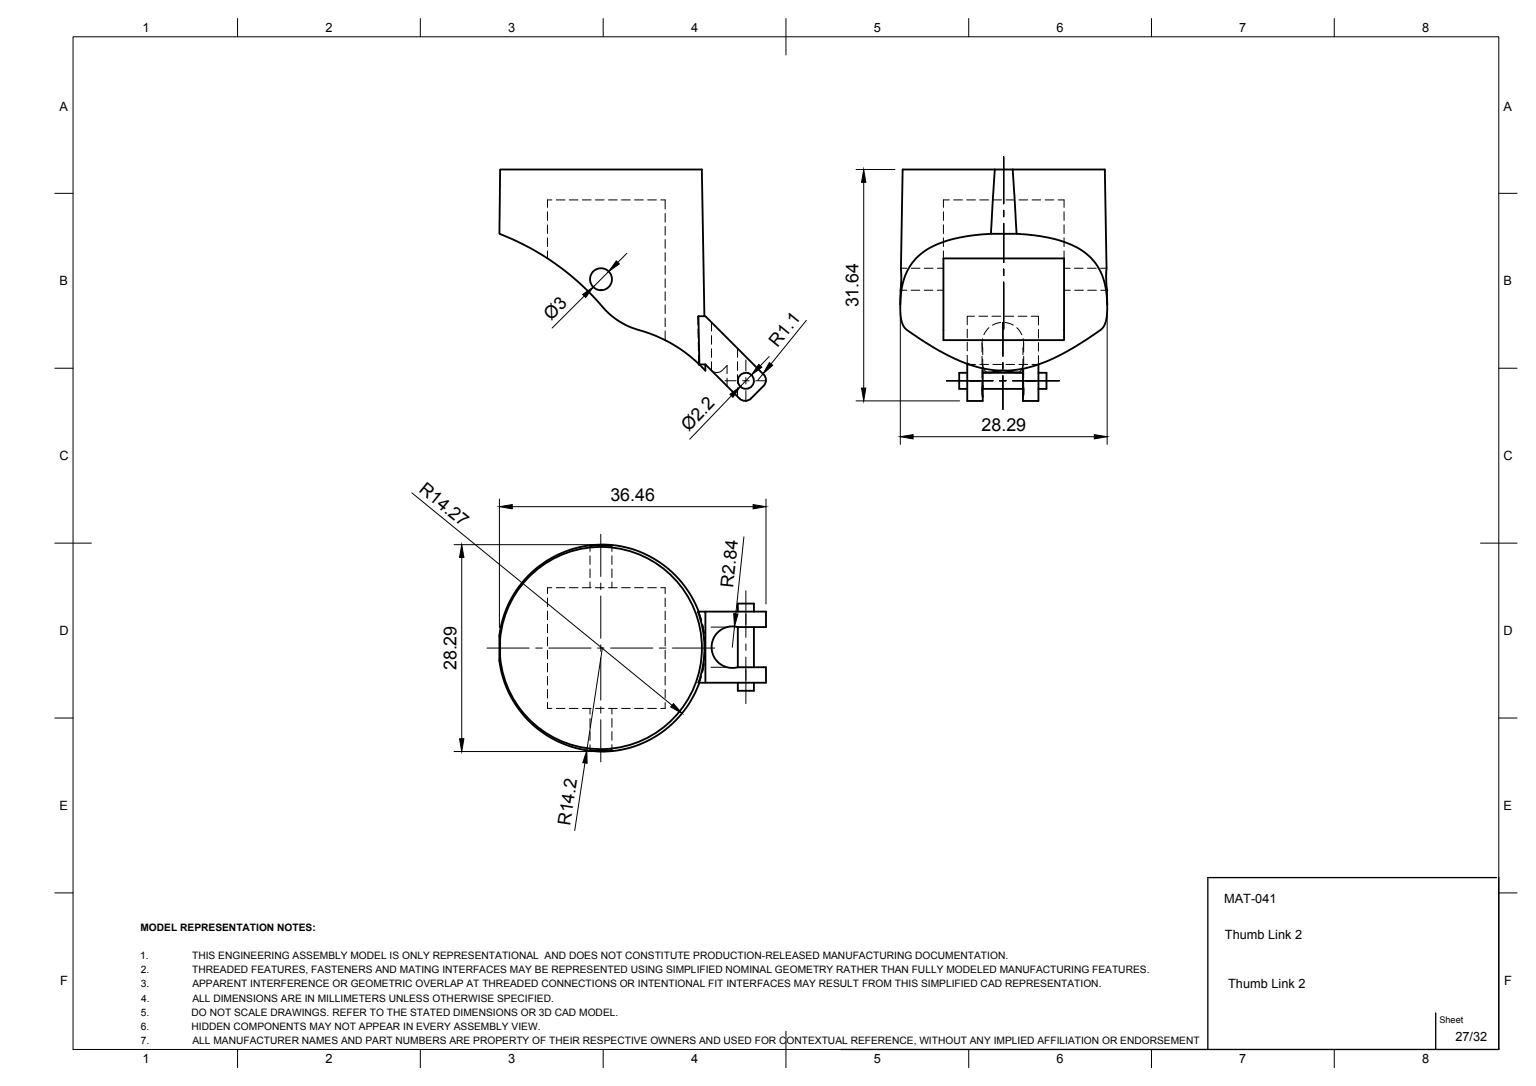
ISO-10303-21;
HEADER;
/* Generated by software containing ST-Developer
 * from STEP Tools, Inc. (www.steptools.com) 
 */

FILE_DESCRIPTION(
/* description */ ('STEP AP214'),
/* implementation_level */ '2;1');

FILE_NAME(
/* name */ 'Thumb Link 2.step',
/* time_stamp */ '2026-11-14T21:57:47-08:00',
/* author */ (''),
/* organization */ (''),
/* preprocessor_version */ 'ST-DEVELOPER v20.2',
/* originating_system */ 'Autodesk Translation Framework v15.17.0.0',
/* authorisation */ '');

FILE_SCHEMA (('AUTOMOTIVE_DESIGN { 1 0 10303 214 3 1 1 }'));
ENDSEC;

DATA;
#10=MECHANICAL_DESIGN_GEOMETRIC_PRESENTATION_REPRESENTATION('',(#262),#13199);
#14=(
BOUNDED_CURVE()
B_SPLINE_CURVE(2,(#12779,#12780,#12781),.UNSPECIFIED.,.F.,.F.)
B_SPLINE_CURVE_WITH_KNOTS((3,3),(-2.71364129597392,-1.62020359036119),
 .UNSPECIFIED.)
CURVE()
GEOMETRIC_REPRESENTATION_ITEM()
RATIONAL_B_SPLINE_CURVE((1.0005626059293,1.00242625759818,1.00269667985146))
REPRESENTATION_ITEM('')
);
#15=(
BOUNDED_CURVE()
B_SPLINE_CURVE(2,(#12785,#12786,#12787),.UNSPECIFIED.,.F.,.F.)
B_SPLINE_CURVE_WITH_KNOTS((3,3),(-1.2490205262323,-0.155582820602816),
 .UNSPECIFIED.)
CURVE()
GEOMETRIC_REPRESENTATION_ITEM()
RATIONAL_B_SPLINE_CURVE((1.00269667985147,1.00242625759819,1.00056260592924))
REPRESENTATION_ITEM('')
);
#16=(
BOUNDED_CURVE()
B_SPLINE_CURVE(2,(#12826,#12827,#12828),.UNSPECIFIED.,.F.,.F.)
B_SPLINE_CURVE_WITH_KNOTS((3,3),(0.587541837462245,1.2406747936684),
 .UNSPECIFIED.)
CURVE()
GEOMETRIC_REPRESENTATION_ITEM()
RATIONAL_B_SPLINE_CURVE((1.00007054095476,1.00010145473128,1.00011392829506))
REPRESENTATION_ITEM('')
);
#124=CONICAL_SURFACE('',#7720,14.3,0.0174532925199433);
#125=CONICAL_SURFACE('',#7729,14.3,0.0174532925199433);
#126=CONICAL_SURFACE('',#7753,14.3,0.0174532925199433);
#199=B_SPLINE_CURVE_WITH_KNOTS('',3,(#12595,#12596,#12597,#12598,#12599,
#12600,#12601,#12602,#12603,#12604,#12605,#12606,#12607,#12608,#12609,#12610,
#12611,#12612,#12613,#12614),.UNSPECIFIED.,.F.,.F.,(4,2,2,2,2,2,2,2,2,4),
(1.13069615346588,1.18716968917911,1.24364799854408,1.30009527290761,1.35654254727113,
1.41319810974912,1.46985367222711,1.526495709458,1.58313774668889,1.58314252031411),
 .UNSPECIFIED.);
#200=B_SPLINE_CURVE_WITH_KNOTS('',3,(#12615,#12616,#12617,#12618,#12619,
#12620,#12621,#12622,#12623,#12624,#12625,#12626,#12627,#12628,#12629,#12630,
#12631,#12632,#12633,#12634,#12635),.UNSPECIFIED.,.F.,.F.,(4,2,2,2,3,2,
2,2,2,4),(0.678287603396378,0.734918137493847,0.791553445216531,0.848204181067131,
0.904854916917731,0.961302354464157,1.01774979201058,1.07422058591236,1.13069137981413,
1.13069615346588),.UNSPECIFIED.);
#201=B_SPLINE_CURVE_WITH_KNOTS('',3,(#12639,#12640,#12641,#12642,#12643,
#12644,#12645,#12646,#12647,#12648,#12649,#12650,#12651,#12652,#12653,#12654,
#12655,#12656,#12657,#12658),.UNSPECIFIED.,.F.,.F.,(4,2,2,2,2,2,2,2,2,4),
(-0.678287603396414,-0.678282829771164,-0.621640792540269,-0.564998755309374,
-0.508343192831388,-0.451687630353401,-0.395240355989875,-0.338793081626349,
-0.282314772261376,-0.225841236548144),.UNSPECIFIED.);
#202=B_SPLINE_CURVE_WITH_KNOTS('',3,(#12662,#12663,#12664,#12665,#12666,
#12667,#12668,#12669,#12670,#12671,#12672,#12673,#12674,#12675,#12676,#12677,
#12678,#12679,#12680,#12681,#12682),.UNSPECIFIED.,.F.,.F.,(4,2,2,2,2,3,
2,2,2,4),(-0.225841236548144,-0.225836462896404,-0.169365668994628,-0.112894875092852,
-0.0564474375464262,0.,0.0566507358506003,0.113301471701201,0.169936779423884,
0.226567313521317),.UNSPECIFIED.);
#203=B_SPLINE_CURVE_WITH_KNOTS('',3,(#12686,#12687,#12688,#12689,#12690,
#12691,#12692,#12693,#12694,#12695,#12696,#12697,#12698,#12699,#12700,#12701,
#12702,#12703),.UNSPECIFIED.,.F.,.F.,(4,2,2,2,2,2,2,2,4),(-0.688543100579729,
-0.654814812371682,-0.585385027074312,-0.486026911248501,-0.386668795422691,
-0.287310679596881,-0.18795256377107,-0.1185227784737,-0.0847944902653396),
 .UNSPECIFIED.);
#204=B_SPLINE_CURVE_WITH_KNOTS('',3,(#12742,#12743,#12744,#12745,#12746,
#12747,#12748,#12749,#12750,#12751),.UNSPECIFIED.,.F.,.F.,(4,2,2,2,4),(2.79683412091131,
2.83278881190682,3.39223982604309,3.96523585047702,4.02795363969691),
 .UNSPECIFIED.);
#205=B_SPLINE_CURVE_WITH_KNOTS('',3,(#12753,#12754,#12755,#12756,#12757,
#12758,#12759,#12760,#12761,#12762),.UNSPECIFIED.,.F.,.F.,(4,2,2,2,4),(10.3179905566208,
10.457151700737,10.6290799698098,10.8010082388826,10.8999538958969),
 .UNSPECIFIED.);
#206=B_SPLINE_CURVE_WITH_KNOTS('',3,(#12764,#12765,#12766,#12767,#12768,
#12769,#12770,#12771,#12772,#12773,#12774,#12775,#12776,#12777),
 .UNSPECIFIED.,.F.,.F.,(4,2,2,2,2,2,4),(-7.02551957351303,-6.83439163802274,
-6.07684267508665,-5.67712314178527,-5.27740360848388,-4.91546143594968,
-4.72326894801671),.UNSPECIFIED.);
#207=B_SPLINE_CURVE_WITH_KNOTS('',3,(#12789,#12790,#12791,#12792,#12793,
#12794,#12795,#12796,#12797,#12798,#12799,#12800,#12801,#12802),
 .UNSPECIFIED.,.F.,.F.,(4,2,2,2,2,2,4),(-4.38376957881428,-4.1915770908813,
-3.82963491834711,-3.42991538504572,-3.03019585174433,-2.27264688880825,
-2.08151895331795),.UNSPECIFIED.);
#208=B_SPLINE_CURVE_WITH_KNOTS('',3,(#12804,#12805,#12806,#12807,#12808,
#12809,#12810,#12811,#12812,#12813),.UNSPECIFIED.,.F.,.F.,(4,2,2,2,4),(6.41116921174888,
6.5101148687632,6.68204313783601,6.85397140690883,6.993132551025),
 .UNSPECIFIED.);
#209=B_SPLINE_CURVE_WITH_KNOTS('',3,(#12815,#12816,#12817,#12818,#12819,
#12820,#12821,#12822,#12823,#12824),.UNSPECIFIED.,.F.,.F.,(4,2,2,2,4),(5.02250397090605,
5.11122789934489,5.68422392377882,6.24367493791509,6.2796296289106),
 .UNSPECIFIED.);
#210=B_SPLINE_CURVE_WITH_KNOTS('',3,(#12831,#12832,#12833,#12834,#12835),
 .UNSPECIFIED.,.F.,.F.,(4,1,4),(0.0247143916721011,0.0279654930527155,0.0312302909052024),
 .UNSPECIFIED.);
#211=B_SPLINE_CURVE_WITH_KNOTS('',3,(#12862,#12863,#12864,#12865,#12866,
#12867,#12868,#12869,#12870,#12871),.UNSPECIFIED.,.F.,.F.,(4,2,2,2,4),(4.05396350737764,
4.25173386269399,4.53823187491096,4.82472988712792,5.02250024244427),
 .UNSPECIFIED.);
#226=SHAPE_REPRESENTATION_RELATIONSHIP('SRR','None',#13298,#244);
#244=ADVANCED_BREP_SHAPE_REPRESENTATION('',(#280),#13194);
#262=STYLED_ITEM('',(#13409),#280);
#280=MANIFOLD_SOLID_BREP('Body1',#6857);
#368=FACE_BOUND('',#2609,.T.);
#369=FACE_BOUND('',#2610,.T.);
#370=FACE_BOUND('',#2620,.T.);
#371=FACE_BOUND('',#2622,.T.);
#372=FACE_BOUND('',#2626,.T.);
#373=FACE_BOUND('',#2629,.T.);
#374=FACE_BOUND('',#2636,.T.);
#375=FACE_BOUND('',#2638,.T.);
#392=ELLIPSE('',#7706,4.01857269385652,2.84156000250712);
#393=ELLIPSE('',#7707,4.01857269388513,2.84156000253857);
#394=ELLIPSE('',#7708,4.01857269388335,2.841560002536);
#395=ELLIPSE('',#7709,4.01857269388599,2.84156000253982);
#396=ELLIPSE('',#7710,4.01857269402875,2.84156000270659);
#573=PLANE('',#7723);
#574=PLANE('',#7724);
#575=PLANE('',#7726);
#576=PLANE('',#7728);
#577=PLANE('',#7735);
#578=PLANE('',#7736);
#579=PLANE('',#7737);
#580=PLANE('',#7740);
#581=PLANE('',#7743);
#582=PLANE('',#7744);
#583=PLANE('',#7746);
#584=PLANE('',#7749);
#585=PLANE('',#7750);
#586=PLANE('',#7754);
#587=PLANE('',#7755);
#588=PLANE('',#7756);
#589=PLANE('',#7757);
#590=PLANE('',#7758);
#591=PLANE('',#7761);
#592=PLANE('',#7764);
#593=PLANE('',#7765);
#594=PLANE('',#7772);
#595=PLANE('',#7773);
#1044=LINE('',#12593,#1562);
#1045=LINE('',#12660,#1563);
#1046=LINE('',#12707,#1564);
#1047=LINE('',#12711,#1565);
#1048=LINE('',#12715,#1566);
#1049=LINE('',#12719,#1567);
#1050=LINE('',#12725,#1568);
#1051=LINE('',#12731,#1569);
#1052=LINE('',#12737,#1570);
#1053=LINE('',#12838,#1571);
#1054=LINE('',#12839,#1572);
#1055=LINE('',#12842,#1573);
#1056=LINE('',#12846,#1574);
#1057=LINE('',#12848,#1575);
#1058=LINE('',#12853,#1576);
#1059=LINE('',#12855,#1577);
#1060=LINE('',#12857,#1578);
#1061=LINE('',#12858,#1579);
#1062=LINE('',#12876,#1580);
#1063=LINE('',#12879,#1581);
#1064=LINE('',#12882,#1582);
#1065=LINE('',#12884,#1583);
#1066=LINE('',#12885,#1584);
#1067=LINE('',#12893,#1585);
#1068=LINE('',#12895,#1586);
#1069=LINE('',#12896,#1587);
#1070=LINE('',#12903,#1588);
#1071=LINE('',#12905,#1589);
#1072=LINE('',#12906,#1590);
#1073=LINE('',#12908,#1591);
#1074=LINE('',#12913,#1592);
#1075=LINE('',#12915,#1593);
#1076=LINE('',#12916,#1594);
#1077=LINE('',#12920,#1595);
#1078=LINE('',#12924,#1596);
#1079=LINE('',#12925,#1597);
#1080=LINE('',#12927,#1598);
#1081=LINE('',#12931,#1599);
#1082=LINE('',#12932,#1600);
#1083=LINE('',#12935,#1601);
#1084=LINE('',#12939,#1602);
#1085=LINE('',#12940,#1603);
#1086=LINE('',#12944,#1604);
#1087=LINE('',#12945,#1605);
#1088=LINE('',#12947,#1606);
#1089=LINE('',#12948,#1607);
#1090=LINE('',#12949,#1608);
#1091=LINE('',#12952,#1609);
#1092=LINE('',#12954,#1610);
#1093=LINE('',#12955,#1611);
#1094=LINE('',#12956,#1612);
#1095=LINE('',#12960,#1613);
#1096=LINE('',#12961,#1614);
#1097=LINE('',#12962,#1615);
#1098=LINE('',#12964,#1616);
#1099=LINE('',#12979,#1617);
#1100=LINE('',#12980,#1618);
#1101=LINE('',#12981,#1619);
#1102=LINE('',#12983,#1620);
#1562=VECTOR('',#9549,1.5);
#1563=VECTOR('',#9552,1.5);
#1564=VECTOR('',#9559,1000.);
#1565=VECTOR('',#9562,1000.);
#1566=VECTOR('',#9565,1000.);
#1567=VECTOR('',#9568,1000.);
#1568=VECTOR('',#9575,1.1);
#1569=VECTOR('',#9582,1.1);
#1570=VECTOR('',#9589,1.1);
#1571=VECTOR('',#9600,1000.);
#1572=VECTOR('',#9601,1000.);
#1573=VECTOR('',#9604,1000.);
#1574=VECTOR('',#9609,1000.);
#1575=VECTOR('',#9610,1000.);
#1576=VECTOR('',#9615,1000.);
#1577=VECTOR('',#9616,1000.);
#1578=VECTOR('',#9617,1000.);
#1579=VECTOR('',#9618,1000.);
#1580=VECTOR('',#9627,1000.);
#1581=VECTOR('',#9630,1000.);
#1582=VECTOR('',#9633,1000.);
#1583=VECTOR('',#9636,1000.);
#1584=VECTOR('',#9637,1000.);
#1585=VECTOR('',#9646,1000.);
#1586=VECTOR('',#9647,1000.);
#1587=VECTOR('',#9648,1000.);
#1588=VECTOR('',#9655,1000.);
#1589=VECTOR('',#9656,1000.);
#1590=VECTOR('',#9657,1000.);
#1591=VECTOR('',#9660,1000.);
#1592=VECTOR('',#9665,1000.);
#1593=VECTOR('',#9666,1000.);
#1594=VECTOR('',#9667,1000.);
#1595=VECTOR('',#9670,1000.);
#1596=VECTOR('',#9673,1000.);
#1597=VECTOR('',#9674,1000.);
#1598=VECTOR('',#9675,1000.);
#1599=VECTOR('',#9680,1000.);
#1600=VECTOR('',#9681,1000.);
#1601=VECTOR('',#9684,1000.);
#1602=VECTOR('',#9689,1000.);
#1603=VECTOR('',#9690,10.);
#1604=VECTOR('',#9695,1000.);
#1605=VECTOR('',#9696,1000.);
#1606=VECTOR('',#9697,1000.);
#1607=VECTOR('',#9698,1000.);
#1608=VECTOR('',#9699,1000.);
#1609=VECTOR('',#9702,1000.);
#1610=VECTOR('',#9703,1000.);
#1611=VECTOR('',#9704,1000.);
#1612=VECTOR('',#9705,1000.);
#1613=VECTOR('',#9708,1000.);
#1614=VECTOR('',#9709,1000.);
#1615=VECTOR('',#9710,1000.);
#1616=VECTOR('',#9713,1000.);
#1617=VECTOR('',#9742,1000.);
#1618=VECTOR('',#9743,1000.);
#1619=VECTOR('',#9744,1000.);
#1620=VECTOR('',#9747,1000.);
#1767=CYLINDRICAL_SURFACE('',#7701,1.5);
#1768=CYLINDRICAL_SURFACE('',#7703,1.5);
#1769=CYLINDRICAL_SURFACE('',#7705,2.84156000253601);
#1770=CYLINDRICAL_SURFACE('',#7711,1.1);
#1771=CYLINDRICAL_SURFACE('',#7714,1.1);
#1772=CYLINDRICAL_SURFACE('',#7717,1.1);
#1773=CYLINDRICAL_SURFACE('',#7731,19.25);
#1774=CYLINDRICAL_SURFACE('',#7766,1.1);
#1775=CYLINDRICAL_SURFACE('',#7767,1.1);
#1776=CYLINDRICAL_SURFACE('',#7768,1.1);
#1777=CYLINDRICAL_SURFACE('',#7769,1.1);
#1778=CYLINDRICAL_SURFACE('',#7770,1.1);
#1779=CYLINDRICAL_SURFACE('',#7771,35.0622035609646);
#1780=CYLINDRICAL_SURFACE('',#7774,10.);
#1781=CYLINDRICAL_SURFACE('',#7775,10.);
#2127=FACE_OUTER_BOUND('',#2602,.T.);
#2128=FACE_OUTER_BOUND('',#2603,.T.);
#2129=FACE_OUTER_BOUND('',#2604,.T.);
#2130=FACE_OUTER_BOUND('',#2605,.T.);
#2131=FACE_OUTER_BOUND('',#2606,.T.);
#2132=FACE_OUTER_BOUND('',#2607,.T.);
#2133=FACE_OUTER_BOUND('',#2608,.T.);
#2134=FACE_OUTER_BOUND('',#2611,.T.);
#2135=FACE_OUTER_BOUND('',#2612,.T.);
#2136=FACE_OUTER_BOUND('',#2613,.T.);
#2137=FACE_OUTER_BOUND('',#2614,.T.);
#2138=FACE_OUTER_BOUND('',#2615,.T.);
#2139=FACE_OUTER_BOUND('',#2616,.T.);
#2140=FACE_OUTER_BOUND('',#2617,.T.);
#2141=FACE_OUTER_BOUND('',#2618,.T.);
#2142=FACE_OUTER_BOUND('',#2619,.T.);
#2143=FACE_OUTER_BOUND('',#2621,.T.);
#2144=FACE_OUTER_BOUND('',#2623,.T.);
#2145=FACE_OUTER_BOUND('',#2624,.T.);
#2146=FACE_OUTER_BOUND('',#2625,.T.);
#2147=FACE_OUTER_BOUND('',#2627,.T.);
#2148=FACE_OUTER_BOUND('',#2628,.T.);
#2149=FACE_OUTER_BOUND('',#2630,.T.);
#2150=FACE_OUTER_BOUND('',#2631,.T.);
#2151=FACE_OUTER_BOUND('',#2632,.T.);
#2152=FACE_OUTER_BOUND('',#2633,.T.);
#2153=FACE_OUTER_BOUND('',#2634,.T.);
#2154=FACE_OUTER_BOUND('',#2635,.T.);
#2155=FACE_OUTER_BOUND('',#2637,.T.);
#2156=FACE_OUTER_BOUND('',#2639,.T.);
#2157=FACE_OUTER_BOUND('',#2640,.T.);
#2158=FACE_OUTER_BOUND('',#2641,.T.);
#2159=FACE_OUTER_BOUND('',#2642,.T.);
#2160=FACE_OUTER_BOUND('',#2643,.T.);
#2161=FACE_OUTER_BOUND('',#2644,.T.);
#2162=FACE_OUTER_BOUND('',#2645,.T.);
#2163=FACE_OUTER_BOUND('',#2646,.T.);
#2164=FACE_OUTER_BOUND('',#2647,.T.);
#2165=FACE_OUTER_BOUND('',#2648,.T.);
#2166=FACE_OUTER_BOUND('',#2649,.T.);
#2167=FACE_OUTER_BOUND('',#2650,.T.);
#2602=EDGE_LOOP('',(#6138,#6139,#6140,#6141,#6142));
#2603=EDGE_LOOP('',(#6143,#6144,#6145,#6146,#6147));
#2604=EDGE_LOOP('',(#6148,#6149,#6150,#6151,#6152,#6153,#6154,#6155,#6156,
#6157));
#2605=EDGE_LOOP('',(#6158,#6159,#6160,#6161));
#2606=EDGE_LOOP('',(#6162,#6163,#6164,#6165));
#2607=EDGE_LOOP('',(#6166,#6167,#6168,#6169));
#2608=EDGE_LOOP('',(#6170,#6171,#6172,#6173,#6174,#6175,#6176,#6177,#6178,
#6179,#6180,#6181));
#2609=EDGE_LOOP('',(#6182,#6183));
#2610=EDGE_LOOP('',(#6184,#6185));
#2611=EDGE_LOOP('',(#6186,#6187,#6188));
#2612=EDGE_LOOP('',(#6189,#6190,#6191,#6192));
#2613=EDGE_LOOP('',(#6193,#6194,#6195,#6196));
#2614=EDGE_LOOP('',(#6197,#6198,#6199,#6200));
#2615=EDGE_LOOP('',(#6201,#6202));
#2616=EDGE_LOOP('',(#6203,#6204,#6205,#6206,#6207,#6208,#6209,#6210,#6211));
#2617=EDGE_LOOP('',(#6212,#6213,#6214,#6215));
#2618=EDGE_LOOP('',(#6216,#6217));
#2619=EDGE_LOOP('',(#6218,#6219,#6220,#6221,#6222,#6223));
#2620=EDGE_LOOP('',(#6224));
#2621=EDGE_LOOP('',(#6225,#6226,#6227,#6228,#6229,#6230));
#2622=EDGE_LOOP('',(#6231));
#2623=EDGE_LOOP('',(#6232,#6233,#6234,#6235));
#2624=EDGE_LOOP('',(#6236,#6237,#6238,#6239,#6240));
#2625=EDGE_LOOP('',(#6241,#6242,#6243,#6244,#6245,#6246,#6247,#6248));
#2626=EDGE_LOOP('',(#6249));
#2627=EDGE_LOOP('',(#6250,#6251,#6252,#6253));
#2628=EDGE_LOOP('',(#6254,#6255,#6256,#6257,#6258,#6259,#6260,#6261,#6262));
#2629=EDGE_LOOP('',(#6263));
#2630=EDGE_LOOP('',(#6264,#6265,#6266));
#2631=EDGE_LOOP('',(#6267,#6268,#6269,#6270,#6271,#6272,#6273,#6274,#6275,
#6276,#6277,#6278));
#2632=EDGE_LOOP('',(#6279,#6280,#6281,#6282,#6283,#6284,#6285,#6286));
#2633=EDGE_LOOP('',(#6287,#6288,#6289,#6290));
#2634=EDGE_LOOP('',(#6291,#6292,#6293));
#2635=EDGE_LOOP('',(#6294,#6295,#6296,#6297,#6298,#6299));
#2636=EDGE_LOOP('',(#6300));
#2637=EDGE_LOOP('',(#6301,#6302,#6303,#6304,#6305,#6306));
#2638=EDGE_LOOP('',(#6307));
#2639=EDGE_LOOP('',(#6308));
#2640=EDGE_LOOP('',(#6309));
#2641=EDGE_LOOP('',(#6310,#6311,#6312,#6313));
#2642=EDGE_LOOP('',(#6314,#6315,#6316,#6317));
#2643=EDGE_LOOP('',(#6318,#6319,#6320,#6321));
#2644=EDGE_LOOP('',(#6322,#6323,#6324,#6325));
#2645=EDGE_LOOP('',(#6326,#6327,#6328,#6329,#6330,#6331));
#2646=EDGE_LOOP('',(#6332,#6333,#6334,#6335,#6336,#6337,#6338,#6339));
#2647=EDGE_LOOP('',(#6340,#6341,#6342,#6343));
#2648=EDGE_LOOP('',(#6344,#6345,#6346,#6347));
#2649=EDGE_LOOP('',(#6348,#6349,#6350,#6351));
#2650=EDGE_LOOP('',(#6352,#6353,#6354,#6355));
#2953=CIRCLE('',#7702,1.5);
#2954=CIRCLE('',#7704,1.5);
#2955=CIRCLE('',#7712,1.1);
#2956=CIRCLE('',#7713,1.1);
#2957=CIRCLE('',#7715,1.1);
#2958=CIRCLE('',#7716,1.1);
#2959=CIRCLE('',#7718,1.1);
#2960=CIRCLE('',#7719,1.1);
#2961=CIRCLE('',#7721,13.819985714474);
#2962=CIRCLE('',#7722,14.1700407574314);
#2963=CIRCLE('',#7725,1.1);
#2964=CIRCLE('',#7727,1.1);
#2965=CIRCLE('',#7730,14.2852441859577);
#2966=CIRCLE('',#7732,19.25);
#2967=CIRCLE('',#7733,13.243680107935);
#2968=CIRCLE('',#7734,19.25);
#2969=CIRCLE('',#7738,35.0622035609646);
#2970=CIRCLE('',#7739,10.);
#2971=CIRCLE('',#7741,10.);
#2972=CIRCLE('',#7742,35.0622035609646);
#2973=CIRCLE('',#7745,14.2852441859577);
#2974=CIRCLE('',#7747,1.1);
#2975=CIRCLE('',#7748,1.1);
#2976=CIRCLE('',#7751,1.1);
#2977=CIRCLE('',#7752,1.1);
#2978=CIRCLE('',#7759,1.1);
#2979=CIRCLE('',#7760,1.1);
#2980=CIRCLE('',#7762,1.1);
#2981=CIRCLE('',#7763,1.1);
#3515=VERTEX_POINT('',#12590);
#3516=VERTEX_POINT('',#12592);
#3517=VERTEX_POINT('',#12594);
#3518=VERTEX_POINT('',#12637);
#3519=VERTEX_POINT('',#12638);
#3520=VERTEX_POINT('',#12659);
#3521=VERTEX_POINT('',#12684);
#3522=VERTEX_POINT('',#12685);
#3523=VERTEX_POINT('',#12704);
#3524=VERTEX_POINT('',#12706);
#3525=VERTEX_POINT('',#12708);
#3526=VERTEX_POINT('',#12710);
#3527=VERTEX_POINT('',#12712);
#3528=VERTEX_POINT('',#12714);
#3529=VERTEX_POINT('',#12716);
#3530=VERTEX_POINT('',#12718);
#3531=VERTEX_POINT('',#12722);
#3532=VERTEX_POINT('',#12724);
#3533=VERTEX_POINT('',#12728);
#3534=VERTEX_POINT('',#12730);
#3535=VERTEX_POINT('',#12734);
#3536=VERTEX_POINT('',#12736);
#3537=VERTEX_POINT('',#12740);
#3538=VERTEX_POINT('',#12741);
#3539=VERTEX_POINT('',#12752);
#3540=VERTEX_POINT('',#12763);
#3541=VERTEX_POINT('',#12778);
#3542=VERTEX_POINT('',#12782);
#3543=VERTEX_POINT('',#12784);
#3544=VERTEX_POINT('',#12788);
#3545=VERTEX_POINT('',#12803);
#3546=VERTEX_POINT('',#12814);
#3547=VERTEX_POINT('',#12825);
#3548=VERTEX_POINT('',#12829);
#3549=VERTEX_POINT('',#12837);
#3550=VERTEX_POINT('',#12841);
#3551=VERTEX_POINT('',#12845);
#3552=VERTEX_POINT('',#12847);
#3553=VERTEX_POINT('',#12851);
#3554=VERTEX_POINT('',#12852);
#3555=VERTEX_POINT('',#12854);
#3556=VERTEX_POINT('',#12856);
#3557=VERTEX_POINT('',#12860);
#3558=VERTEX_POINT('',#12873);
#3559=VERTEX_POINT('',#12874);
#3560=VERTEX_POINT('',#12878);
#3561=VERTEX_POINT('',#12880);
#3562=VERTEX_POINT('',#12888);
#3563=VERTEX_POINT('',#12889);
#3564=VERTEX_POINT('',#12892);
#3565=VERTEX_POINT('',#12894);
#3566=VERTEX_POINT('',#12898);
#3567=VERTEX_POINT('',#12900);
#3568=VERTEX_POINT('',#12902);
#3569=VERTEX_POINT('',#12904);
#3570=VERTEX_POINT('',#12910);
#3571=VERTEX_POINT('',#12912);
#3572=VERTEX_POINT('',#12914);
#3573=VERTEX_POINT('',#12918);
#3574=VERTEX_POINT('',#12919);
#3575=VERTEX_POINT('',#12921);
#3576=VERTEX_POINT('',#12923);
#3577=VERTEX_POINT('',#12926);
#3578=VERTEX_POINT('',#12930);
#3579=VERTEX_POINT('',#12934);
#3580=VERTEX_POINT('',#12937);
#3581=VERTEX_POINT('',#12943);
#3582=VERTEX_POINT('',#12946);
#3583=VERTEX_POINT('',#12951);
#3584=VERTEX_POINT('',#12953);
#3585=VERTEX_POINT('',#12958);
#3586=VERTEX_POINT('',#12959);
#4406=EDGE_CURVE('',#3515,#3515,#2953,.T.);
#4407=EDGE_CURVE('',#3515,#3516,#1044,.T.);
#4408=EDGE_CURVE('',#3516,#3517,#199,.T.);
#4409=EDGE_CURVE('',#3517,#3516,#200,.T.);
#4410=EDGE_CURVE('',#3518,#3519,#201,.T.);
#4411=EDGE_CURVE('',#3519,#3520,#1045,.T.);
#4412=EDGE_CURVE('',#3520,#3520,#2954,.T.);
#4413=EDGE_CURVE('',#3519,#3518,#202,.T.);
#4414=EDGE_CURVE('',#3521,#3522,#203,.T.);
#4415=EDGE_CURVE('',#3523,#3522,#392,.T.);
#4416=EDGE_CURVE('',#3524,#3523,#1046,.T.);
#4417=EDGE_CURVE('',#3525,#3524,#393,.T.);
#4418=EDGE_CURVE('',#3525,#3526,#1047,.T.);
#4419=EDGE_CURVE('',#3527,#3526,#394,.T.);
#4420=EDGE_CURVE('',#3528,#3527,#1048,.T.);
#4421=EDGE_CURVE('',#3529,#3528,#395,.T.);
#4422=EDGE_CURVE('',#3530,#3529,#1049,.T.);
#4423=EDGE_CURVE('',#3521,#3530,#396,.T.);
#4424=EDGE_CURVE('',#3531,#3531,#2955,.T.);
#4425=EDGE_CURVE('',#3531,#3532,#1050,.T.);
#4426=EDGE_CURVE('',#3532,#3532,#2956,.T.);
#4427=EDGE_CURVE('',#3533,#3533,#2957,.T.);
#4428=EDGE_CURVE('',#3533,#3534,#1051,.T.);
#4429=EDGE_CURVE('',#3534,#3534,#2958,.T.);
#4430=EDGE_CURVE('',#3535,#3535,#2959,.T.);
#4431=EDGE_CURVE('',#3535,#3536,#1052,.T.);
#4432=EDGE_CURVE('',#3536,#3536,#2960,.T.);
#4433=EDGE_CURVE('',#3537,#3538,#204,.T.);
#4434=EDGE_CURVE('',#3537,#3539,#205,.T.);
#4435=EDGE_CURVE('',#3539,#3540,#206,.T.);
#4436=EDGE_CURVE('',#3541,#3540,#14,.T.);
#4437=EDGE_CURVE('',#3542,#3541,#2961,.T.);
#4438=EDGE_CURVE('',#3543,#3542,#15,.T.);
#4439=EDGE_CURVE('',#3543,#3544,#207,.T.);
#4440=EDGE_CURVE('',#3544,#3545,#208,.T.);
#4441=EDGE_CURVE('',#3546,#3545,#209,.T.);
#4442=EDGE_CURVE('',#3546,#3547,#16,.T.);
#4443=EDGE_CURVE('',#3547,#3548,#2962,.T.);
#4444=EDGE_CURVE('',#3548,#3538,#210,.T.);
#4445=EDGE_CURVE('',#3549,#3523,#1053,.T.);
#4446=EDGE_CURVE('',#3522,#3549,#1054,.T.);
#4447=EDGE_CURVE('',#3524,#3550,#1055,.T.);
#4448=EDGE_CURVE('',#3549,#3550,#2963,.T.);
#4449=EDGE_CURVE('',#3551,#3530,#1056,.T.);
#4450=EDGE_CURVE('',#3552,#3529,#1057,.T.);
#4451=EDGE_CURVE('',#3552,#3551,#2964,.T.);
#4452=EDGE_CURVE('',#3553,#3554,#1058,.T.);
#4453=EDGE_CURVE('',#3554,#3555,#1059,.T.);
#4454=EDGE_CURVE('',#3556,#3555,#1060,.T.);
#4455=EDGE_CURVE('',#3556,#3553,#1061,.T.);
#4456=EDGE_CURVE('',#3557,#3546,#2965,.T.);
#4457=EDGE_CURVE('',#3557,#3546,#211,.T.);
#4458=EDGE_CURVE('',#3558,#3559,#2966,.T.);
#4459=EDGE_CURVE('',#3559,#3537,#1062,.T.);
#4460=EDGE_CURVE('',#3538,#3557,#2967,.T.);
#4461=EDGE_CURVE('',#3545,#3560,#1063,.T.);
#4462=EDGE_CURVE('',#3560,#3561,#2968,.T.);
#4463=EDGE_CURVE('',#3558,#3561,#1064,.T.);
#4464=EDGE_CURVE('',#3543,#3540,#1065,.T.);
#4465=EDGE_CURVE('',#3541,#3542,#1066,.T.);
#4466=EDGE_CURVE('',#3562,#3563,#2969,.T.);
#4467=EDGE_CURVE('',#3562,#3559,#2970,.T.);
#4468=EDGE_CURVE('',#3564,#3558,#1067,.T.);
#4469=EDGE_CURVE('',#3565,#3564,#1068,.T.);
#4470=EDGE_CURVE('',#3565,#3563,#1069,.T.);
#4471=EDGE_CURVE('',#3560,#3566,#2971,.T.);
#4472=EDGE_CURVE('',#3567,#3566,#2972,.T.);
#4473=EDGE_CURVE('',#3568,#3567,#1070,.T.);
#4474=EDGE_CURVE('',#3569,#3568,#1071,.T.);
#4475=EDGE_CURVE('',#3561,#3569,#1072,.T.);
#4476=EDGE_CURVE('',#3564,#3569,#1073,.T.);
#4477=EDGE_CURVE('',#3570,#3557,#2973,.T.);
#4478=EDGE_CURVE('',#3570,#3571,#1074,.T.);
#4479=EDGE_CURVE('',#3571,#3572,#1075,.T.);
#4480=EDGE_CURVE('',#3546,#3572,#1076,.T.);
#4481=EDGE_CURVE('',#3573,#3574,#1077,.T.);
#4482=EDGE_CURVE('',#3573,#3575,#2974,.T.);
#4483=EDGE_CURVE('',#3575,#3576,#1078,.T.);
#4484=EDGE_CURVE('',#3547,#3576,#1079,.T.);
#4485=EDGE_CURVE('',#3577,#3572,#1080,.T.);
#4486=EDGE_CURVE('',#3577,#3574,#2975,.T.);
#4487=EDGE_CURVE('',#3576,#3578,#1081,.T.);
#4488=EDGE_CURVE('',#3548,#3578,#1082,.T.);
#4489=EDGE_CURVE('',#3579,#3578,#1083,.T.);
#4490=EDGE_CURVE('',#3579,#3554,#2976,.T.);
#4491=EDGE_CURVE('',#3553,#3580,#2977,.T.);
#4492=EDGE_CURVE('',#3580,#3571,#1084,.T.);
#4493=EDGE_CURVE('',#3538,#3570,#1085,.T.);
#4494=EDGE_CURVE('',#3528,#3581,#1086,.T.);
#4495=EDGE_CURVE('',#3581,#3577,#1087,.T.);
#4496=EDGE_CURVE('',#3580,#3582,#1088,.T.);
#4497=EDGE_CURVE('',#3582,#3525,#1089,.T.);
#4498=EDGE_CURVE('',#3550,#3552,#1090,.T.);
#4499=EDGE_CURVE('',#3527,#3583,#1091,.T.);
#4500=EDGE_CURVE('',#3584,#3526,#1092,.T.);
#4501=EDGE_CURVE('',#3584,#3579,#1093,.T.);
#4502=EDGE_CURVE('',#3575,#3583,#1094,.T.);
#4503=EDGE_CURVE('',#3585,#3586,#1095,.T.);
#4504=EDGE_CURVE('',#3585,#3573,#1096,.T.);
#4505=EDGE_CURVE('',#3574,#3586,#1097,.T.);
#4506=EDGE_CURVE('',#3551,#3521,#1098,.T.);
#4507=EDGE_CURVE('',#3582,#3556,#2978,.T.);
#4508=EDGE_CURVE('',#3555,#3584,#2979,.T.);
#4509=EDGE_CURVE('',#3583,#3585,#2980,.T.);
#4510=EDGE_CURVE('',#3586,#3581,#2981,.T.);
#4511=EDGE_CURVE('',#3539,#3562,#1099,.T.);
#4512=EDGE_CURVE('',#3563,#3567,#1100,.T.);
#4513=EDGE_CURVE('',#3566,#3544,#1101,.T.);
#4514=EDGE_CURVE('',#3568,#3565,#1102,.T.);
#6138=ORIENTED_EDGE('',*,*,#4406,.F.);
#6139=ORIENTED_EDGE('',*,*,#4407,.T.);
#6140=ORIENTED_EDGE('',*,*,#4408,.T.);
#6141=ORIENTED_EDGE('',*,*,#4409,.T.);
#6142=ORIENTED_EDGE('',*,*,#4407,.F.);
#6143=ORIENTED_EDGE('',*,*,#4410,.T.);
#6144=ORIENTED_EDGE('',*,*,#4411,.T.);
#6145=ORIENTED_EDGE('',*,*,#4412,.F.);
#6146=ORIENTED_EDGE('',*,*,#4411,.F.);
#6147=ORIENTED_EDGE('',*,*,#4413,.T.);
#6148=ORIENTED_EDGE('',*,*,#4414,.T.);
#6149=ORIENTED_EDGE('',*,*,#4415,.F.);
#6150=ORIENTED_EDGE('',*,*,#4416,.F.);
#6151=ORIENTED_EDGE('',*,*,#4417,.F.);
#6152=ORIENTED_EDGE('',*,*,#4418,.T.);
#6153=ORIENTED_EDGE('',*,*,#4419,.F.);
#6154=ORIENTED_EDGE('',*,*,#4420,.F.);
#6155=ORIENTED_EDGE('',*,*,#4421,.F.);
#6156=ORIENTED_EDGE('',*,*,#4422,.F.);
#6157=ORIENTED_EDGE('',*,*,#4423,.F.);
#6158=ORIENTED_EDGE('',*,*,#4424,.T.);
#6159=ORIENTED_EDGE('',*,*,#4425,.T.);
#6160=ORIENTED_EDGE('',*,*,#4426,.T.);
#6161=ORIENTED_EDGE('',*,*,#4425,.F.);
#6162=ORIENTED_EDGE('',*,*,#4427,.T.);
#6163=ORIENTED_EDGE('',*,*,#4428,.T.);
#6164=ORIENTED_EDGE('',*,*,#4429,.F.);
#6165=ORIENTED_EDGE('',*,*,#4428,.F.);
#6166=ORIENTED_EDGE('',*,*,#4430,.T.);
#6167=ORIENTED_EDGE('',*,*,#4431,.T.);
#6168=ORIENTED_EDGE('',*,*,#4432,.T.);
#6169=ORIENTED_EDGE('',*,*,#4431,.F.);
#6170=ORIENTED_EDGE('',*,*,#4433,.F.);
#6171=ORIENTED_EDGE('',*,*,#4434,.T.);
#6172=ORIENTED_EDGE('',*,*,#4435,.T.);
#6173=ORIENTED_EDGE('',*,*,#4436,.F.);
#6174=ORIENTED_EDGE('',*,*,#4437,.F.);
#6175=ORIENTED_EDGE('',*,*,#4438,.F.);
#6176=ORIENTED_EDGE('',*,*,#4439,.T.);
#6177=ORIENTED_EDGE('',*,*,#4440,.T.);
#6178=ORIENTED_EDGE('',*,*,#4441,.F.);
#6179=ORIENTED_EDGE('',*,*,#4442,.T.);
#6180=ORIENTED_EDGE('',*,*,#4443,.T.);
#6181=ORIENTED_EDGE('',*,*,#4444,.T.);
#6182=ORIENTED_EDGE('',*,*,#4410,.F.);
#6183=ORIENTED_EDGE('',*,*,#4413,.F.);
#6184=ORIENTED_EDGE('',*,*,#4409,.F.);
#6185=ORIENTED_EDGE('',*,*,#4408,.F.);
#6186=ORIENTED_EDGE('',*,*,#4445,.T.);
#6187=ORIENTED_EDGE('',*,*,#4415,.T.);
#6188=ORIENTED_EDGE('',*,*,#4446,.T.);
#6189=ORIENTED_EDGE('',*,*,#4447,.F.);
#6190=ORIENTED_EDGE('',*,*,#4416,.T.);
#6191=ORIENTED_EDGE('',*,*,#4445,.F.);
#6192=ORIENTED_EDGE('',*,*,#4448,.T.);
#6193=ORIENTED_EDGE('',*,*,#4449,.T.);
#6194=ORIENTED_EDGE('',*,*,#4422,.T.);
#6195=ORIENTED_EDGE('',*,*,#4450,.F.);
#6196=ORIENTED_EDGE('',*,*,#4451,.T.);
#6197=ORIENTED_EDGE('',*,*,#4452,.T.);
#6198=ORIENTED_EDGE('',*,*,#4453,.T.);
#6199=ORIENTED_EDGE('',*,*,#4454,.F.);
#6200=ORIENTED_EDGE('',*,*,#4455,.T.);
#6201=ORIENTED_EDGE('',*,*,#4456,.T.);
#6202=ORIENTED_EDGE('',*,*,#4457,.F.);
#6203=ORIENTED_EDGE('',*,*,#4458,.T.);
#6204=ORIENTED_EDGE('',*,*,#4459,.T.);
#6205=ORIENTED_EDGE('',*,*,#4433,.T.);
#6206=ORIENTED_EDGE('',*,*,#4460,.T.);
#6207=ORIENTED_EDGE('',*,*,#4457,.T.);
#6208=ORIENTED_EDGE('',*,*,#4441,.T.);
#6209=ORIENTED_EDGE('',*,*,#4461,.T.);
#6210=ORIENTED_EDGE('',*,*,#4462,.T.);
#6211=ORIENTED_EDGE('',*,*,#4463,.F.);
#6212=ORIENTED_EDGE('',*,*,#4464,.F.);
#6213=ORIENTED_EDGE('',*,*,#4438,.T.);
#6214=ORIENTED_EDGE('',*,*,#4465,.F.);
#6215=ORIENTED_EDGE('',*,*,#4436,.T.);
#6216=ORIENTED_EDGE('',*,*,#4437,.T.);
#6217=ORIENTED_EDGE('',*,*,#4465,.T.);
#6218=ORIENTED_EDGE('',*,*,#4466,.F.);
#6219=ORIENTED_EDGE('',*,*,#4467,.T.);
#6220=ORIENTED_EDGE('',*,*,#4458,.F.);
#6221=ORIENTED_EDGE('',*,*,#4468,.F.);
#6222=ORIENTED_EDGE('',*,*,#4469,.F.);
#6223=ORIENTED_EDGE('',*,*,#4470,.T.);
#6224=ORIENTED_EDGE('',*,*,#4406,.T.);
#6225=ORIENTED_EDGE('',*,*,#4462,.F.);
#6226=ORIENTED_EDGE('',*,*,#4471,.T.);
#6227=ORIENTED_EDGE('',*,*,#4472,.F.);
#6228=ORIENTED_EDGE('',*,*,#4473,.F.);
#6229=ORIENTED_EDGE('',*,*,#4474,.F.);
#6230=ORIENTED_EDGE('',*,*,#4475,.F.);
#6231=ORIENTED_EDGE('',*,*,#4412,.T.);
#6232=ORIENTED_EDGE('',*,*,#4463,.T.);
#6233=ORIENTED_EDGE('',*,*,#4475,.T.);
#6234=ORIENTED_EDGE('',*,*,#4476,.F.);
#6235=ORIENTED_EDGE('',*,*,#4468,.T.);
#6236=ORIENTED_EDGE('',*,*,#4477,.F.);
#6237=ORIENTED_EDGE('',*,*,#4478,.T.);
#6238=ORIENTED_EDGE('',*,*,#4479,.T.);
#6239=ORIENTED_EDGE('',*,*,#4480,.F.);
#6240=ORIENTED_EDGE('',*,*,#4456,.F.);
#6241=ORIENTED_EDGE('',*,*,#4481,.F.);
#6242=ORIENTED_EDGE('',*,*,#4482,.T.);
#6243=ORIENTED_EDGE('',*,*,#4483,.T.);
#6244=ORIENTED_EDGE('',*,*,#4484,.F.);
#6245=ORIENTED_EDGE('',*,*,#4442,.F.);
#6246=ORIENTED_EDGE('',*,*,#4480,.T.);
#6247=ORIENTED_EDGE('',*,*,#4485,.F.);
#6248=ORIENTED_EDGE('',*,*,#4486,.T.);
#6249=ORIENTED_EDGE('',*,*,#4426,.F.);
#6250=ORIENTED_EDGE('',*,*,#4443,.F.);
#6251=ORIENTED_EDGE('',*,*,#4484,.T.);
#6252=ORIENTED_EDGE('',*,*,#4487,.T.);
#6253=ORIENTED_EDGE('',*,*,#4488,.F.);
#6254=ORIENTED_EDGE('',*,*,#4489,.F.);
#6255=ORIENTED_EDGE('',*,*,#4490,.T.);
#6256=ORIENTED_EDGE('',*,*,#4452,.F.);
#6257=ORIENTED_EDGE('',*,*,#4491,.T.);
#6258=ORIENTED_EDGE('',*,*,#4492,.T.);
#6259=ORIENTED_EDGE('',*,*,#4478,.F.);
#6260=ORIENTED_EDGE('',*,*,#4493,.F.);
#6261=ORIENTED_EDGE('',*,*,#4444,.F.);
#6262=ORIENTED_EDGE('',*,*,#4488,.T.);
#6263=ORIENTED_EDGE('',*,*,#4427,.F.);
#6264=ORIENTED_EDGE('',*,*,#4477,.T.);
#6265=ORIENTED_EDGE('',*,*,#4460,.F.);
#6266=ORIENTED_EDGE('',*,*,#4493,.T.);
#6267=ORIENTED_EDGE('',*,*,#4450,.T.);
#6268=ORIENTED_EDGE('',*,*,#4421,.T.);
#6269=ORIENTED_EDGE('',*,*,#4494,.T.);
#6270=ORIENTED_EDGE('',*,*,#4495,.T.);
#6271=ORIENTED_EDGE('',*,*,#4485,.T.);
#6272=ORIENTED_EDGE('',*,*,#4479,.F.);
#6273=ORIENTED_EDGE('',*,*,#4492,.F.);
#6274=ORIENTED_EDGE('',*,*,#4496,.T.);
#6275=ORIENTED_EDGE('',*,*,#4497,.T.);
#6276=ORIENTED_EDGE('',*,*,#4417,.T.);
#6277=ORIENTED_EDGE('',*,*,#4447,.T.);
#6278=ORIENTED_EDGE('',*,*,#4498,.T.);
#6279=ORIENTED_EDGE('',*,*,#4499,.F.);
#6280=ORIENTED_EDGE('',*,*,#4419,.T.);
#6281=ORIENTED_EDGE('',*,*,#4500,.F.);
#6282=ORIENTED_EDGE('',*,*,#4501,.T.);
#6283=ORIENTED_EDGE('',*,*,#4489,.T.);
#6284=ORIENTED_EDGE('',*,*,#4487,.F.);
#6285=ORIENTED_EDGE('',*,*,#4483,.F.);
#6286=ORIENTED_EDGE('',*,*,#4502,.T.);
#6287=ORIENTED_EDGE('',*,*,#4503,.F.);
#6288=ORIENTED_EDGE('',*,*,#4504,.T.);
#6289=ORIENTED_EDGE('',*,*,#4481,.T.);
#6290=ORIENTED_EDGE('',*,*,#4505,.T.);
#6291=ORIENTED_EDGE('',*,*,#4506,.T.);
#6292=ORIENTED_EDGE('',*,*,#4423,.T.);
#6293=ORIENTED_EDGE('',*,*,#4449,.F.);
#6294=ORIENTED_EDGE('',*,*,#4500,.T.);
#6295=ORIENTED_EDGE('',*,*,#4418,.F.);
#6296=ORIENTED_EDGE('',*,*,#4497,.F.);
#6297=ORIENTED_EDGE('',*,*,#4507,.T.);
#6298=ORIENTED_EDGE('',*,*,#4454,.T.);
#6299=ORIENTED_EDGE('',*,*,#4508,.T.);
#6300=ORIENTED_EDGE('',*,*,#4432,.F.);
#6301=ORIENTED_EDGE('',*,*,#4494,.F.);
#6302=ORIENTED_EDGE('',*,*,#4420,.T.);
#6303=ORIENTED_EDGE('',*,*,#4499,.T.);
#6304=ORIENTED_EDGE('',*,*,#4509,.T.);
#6305=ORIENTED_EDGE('',*,*,#4503,.T.);
#6306=ORIENTED_EDGE('',*,*,#4510,.T.);
#6307=ORIENTED_EDGE('',*,*,#4430,.F.);
#6308=ORIENTED_EDGE('',*,*,#4429,.T.);
#6309=ORIENTED_EDGE('',*,*,#4424,.F.);
#6310=ORIENTED_EDGE('',*,*,#4509,.F.);
#6311=ORIENTED_EDGE('',*,*,#4502,.F.);
#6312=ORIENTED_EDGE('',*,*,#4482,.F.);
#6313=ORIENTED_EDGE('',*,*,#4504,.F.);
#6314=ORIENTED_EDGE('',*,*,#4490,.F.);
#6315=ORIENTED_EDGE('',*,*,#4501,.F.);
#6316=ORIENTED_EDGE('',*,*,#4508,.F.);
#6317=ORIENTED_EDGE('',*,*,#4453,.F.);
#6318=ORIENTED_EDGE('',*,*,#4507,.F.);
#6319=ORIENTED_EDGE('',*,*,#4496,.F.);
#6320=ORIENTED_EDGE('',*,*,#4491,.F.);
#6321=ORIENTED_EDGE('',*,*,#4455,.F.);
#6322=ORIENTED_EDGE('',*,*,#4486,.F.);
#6323=ORIENTED_EDGE('',*,*,#4495,.F.);
#6324=ORIENTED_EDGE('',*,*,#4510,.F.);
#6325=ORIENTED_EDGE('',*,*,#4505,.F.);
#6326=ORIENTED_EDGE('',*,*,#4414,.F.);
#6327=ORIENTED_EDGE('',*,*,#4506,.F.);
#6328=ORIENTED_EDGE('',*,*,#4451,.F.);
#6329=ORIENTED_EDGE('',*,*,#4498,.F.);
#6330=ORIENTED_EDGE('',*,*,#4448,.F.);
#6331=ORIENTED_EDGE('',*,*,#4446,.F.);
#6332=ORIENTED_EDGE('',*,*,#4435,.F.);
#6333=ORIENTED_EDGE('',*,*,#4511,.T.);
#6334=ORIENTED_EDGE('',*,*,#4466,.T.);
#6335=ORIENTED_EDGE('',*,*,#4512,.T.);
#6336=ORIENTED_EDGE('',*,*,#4472,.T.);
#6337=ORIENTED_EDGE('',*,*,#4513,.T.);
#6338=ORIENTED_EDGE('',*,*,#4439,.F.);
#6339=ORIENTED_EDGE('',*,*,#4464,.T.);
#6340=ORIENTED_EDGE('',*,*,#4512,.F.);
#6341=ORIENTED_EDGE('',*,*,#4470,.F.);
#6342=ORIENTED_EDGE('',*,*,#4514,.F.);
#6343=ORIENTED_EDGE('',*,*,#4473,.T.);
#6344=ORIENTED_EDGE('',*,*,#4474,.T.);
#6345=ORIENTED_EDGE('',*,*,#4514,.T.);
#6346=ORIENTED_EDGE('',*,*,#4469,.T.);
#6347=ORIENTED_EDGE('',*,*,#4476,.T.);
#6348=ORIENTED_EDGE('',*,*,#4434,.F.);
#6349=ORIENTED_EDGE('',*,*,#4459,.F.);
#6350=ORIENTED_EDGE('',*,*,#4467,.F.);
#6351=ORIENTED_EDGE('',*,*,#4511,.F.);
#6352=ORIENTED_EDGE('',*,*,#4471,.F.);
#6353=ORIENTED_EDGE('',*,*,#4461,.F.);
#6354=ORIENTED_EDGE('',*,*,#4440,.F.);
#6355=ORIENTED_EDGE('',*,*,#4513,.F.);
#6779=ADVANCED_FACE('',(#2127),#1767,.F.);
#6780=ADVANCED_FACE('',(#2128),#1768,.F.);
#6781=ADVANCED_FACE('',(#2129),#1769,.F.);
#6782=ADVANCED_FACE('',(#2130),#1770,.T.);
#6783=ADVANCED_FACE('',(#2131),#1771,.T.);
#6784=ADVANCED_FACE('',(#2132),#1772,.T.);
#6785=ADVANCED_FACE('',(#2133,#368,#369),#124,.T.);
#6786=ADVANCED_FACE('',(#2134),#573,.F.);
#6787=ADVANCED_FACE('',(#2135),#574,.F.);
#6788=ADVANCED_FACE('',(#2136),#575,.F.);
#6789=ADVANCED_FACE('',(#2137),#576,.T.);
#6790=ADVANCED_FACE('',(#2138),#125,.T.);
#6791=ADVANCED_FACE('',(#2139),#1773,.F.);
#6792=ADVANCED_FACE('',(#2140),#577,.T.);
#6793=ADVANCED_FACE('',(#2141),#578,.T.);
#6794=ADVANCED_FACE('',(#2142,#370),#579,.T.);
#6795=ADVANCED_FACE('',(#2143,#371),#580,.T.);
#6796=ADVANCED_FACE('',(#2144),#581,.F.);
#6797=ADVANCED_FACE('',(#2145),#582,.F.);
#6798=ADVANCED_FACE('',(#2146,#372),#583,.F.);
#6799=ADVANCED_FACE('',(#2147),#584,.F.);
#6800=ADVANCED_FACE('',(#2148,#373),#585,.F.);
#6801=ADVANCED_FACE('',(#2149),#126,.F.);
#6802=ADVANCED_FACE('',(#2150),#586,.F.);
#6803=ADVANCED_FACE('',(#2151),#587,.F.);
#6804=ADVANCED_FACE('',(#2152),#588,.T.);
#6805=ADVANCED_FACE('',(#2153),#589,.F.);
#6806=ADVANCED_FACE('',(#2154,#374),#590,.F.);
#6807=ADVANCED_FACE('',(#2155,#375),#591,.F.);
#6808=ADVANCED_FACE('',(#2156),#592,.T.);
#6809=ADVANCED_FACE('',(#2157),#593,.F.);
#6810=ADVANCED_FACE('',(#2158),#1774,.T.);
#6811=ADVANCED_FACE('',(#2159),#1775,.T.);
#6812=ADVANCED_FACE('',(#2160),#1776,.T.);
#6813=ADVANCED_FACE('',(#2161),#1777,.T.);
#6814=ADVANCED_FACE('',(#2162),#1778,.T.);
#6815=ADVANCED_FACE('',(#2163),#1779,.F.);
#6816=ADVANCED_FACE('',(#2164),#594,.F.);
#6817=ADVANCED_FACE('',(#2165),#595,.T.);
#6818=ADVANCED_FACE('',(#2166),#1780,.T.);
#6819=ADVANCED_FACE('',(#2167),#1781,.T.);
#6857=CLOSED_SHELL('',(#6779,#6780,#6781,#6782,#6783,#6784,#6785,#6786,
#6787,#6788,#6789,#6790,#6791,#6792,#6793,#6794,#6795,#6796,#6797,#6798,
#6799,#6800,#6801,#6802,#6803,#6804,#6805,#6806,#6807,#6808,#6809,#6810,
#6811,#6812,#6813,#6814,#6815,#6816,#6817,#6818,#6819));
#7700=AXIS2_PLACEMENT_3D('',#12588,#9543,#9544);
#7701=AXIS2_PLACEMENT_3D('',#12589,#9545,#9546);
#7702=AXIS2_PLACEMENT_3D('',#12591,#9547,#9548);
#7703=AXIS2_PLACEMENT_3D('',#12636,#9550,#9551);
#7704=AXIS2_PLACEMENT_3D('',#12661,#9553,#9554);
#7705=AXIS2_PLACEMENT_3D('',#12683,#9555,#9556);
#7706=AXIS2_PLACEMENT_3D('',#12705,#9557,#9558);
#7707=AXIS2_PLACEMENT_3D('',#12709,#9560,#9561);
#7708=AXIS2_PLACEMENT_3D('',#12713,#9563,#9564);
#7709=AXIS2_PLACEMENT_3D('',#12717,#9566,#9567);
#7710=AXIS2_PLACEMENT_3D('',#12720,#9569,#9570);
#7711=AXIS2_PLACEMENT_3D('',#12721,#9571,#9572);
#7712=AXIS2_PLACEMENT_3D('',#12723,#9573,#9574);
#7713=AXIS2_PLACEMENT_3D('',#12726,#9576,#9577);
#7714=AXIS2_PLACEMENT_3D('',#12727,#9578,#9579);
#7715=AXIS2_PLACEMENT_3D('',#12729,#9580,#9581);
#7716=AXIS2_PLACEMENT_3D('',#12732,#9583,#9584);
#7717=AXIS2_PLACEMENT_3D('',#12733,#9585,#9586);
#7718=AXIS2_PLACEMENT_3D('',#12735,#9587,#9588);
#7719=AXIS2_PLACEMENT_3D('',#12738,#9590,#9591);
#7720=AXIS2_PLACEMENT_3D('',#12739,#9592,#9593);
#7721=AXIS2_PLACEMENT_3D('',#12783,#9594,#9595);
#7722=AXIS2_PLACEMENT_3D('',#12830,#9596,#9597);
#7723=AXIS2_PLACEMENT_3D('',#12836,#9598,#9599);
#7724=AXIS2_PLACEMENT_3D('',#12840,#9602,#9603);
#7725=AXIS2_PLACEMENT_3D('',#12843,#9605,#9606);
#7726=AXIS2_PLACEMENT_3D('',#12844,#9607,#9608);
#7727=AXIS2_PLACEMENT_3D('',#12849,#9611,#9612);
#7728=AXIS2_PLACEMENT_3D('',#12850,#9613,#9614);
#7729=AXIS2_PLACEMENT_3D('',#12859,#9619,#9620);
#7730=AXIS2_PLACEMENT_3D('',#12861,#9621,#9622);
#7731=AXIS2_PLACEMENT_3D('',#12872,#9623,#9624);
#7732=AXIS2_PLACEMENT_3D('',#12875,#9625,#9626);
#7733=AXIS2_PLACEMENT_3D('',#12877,#9628,#9629);
#7734=AXIS2_PLACEMENT_3D('',#12881,#9631,#9632);
#7735=AXIS2_PLACEMENT_3D('',#12883,#9634,#9635);
#7736=AXIS2_PLACEMENT_3D('',#12886,#9638,#9639);
#7737=AXIS2_PLACEMENT_3D('',#12887,#9640,#9641);
#7738=AXIS2_PLACEMENT_3D('',#12890,#9642,#9643);
#7739=AXIS2_PLACEMENT_3D('',#12891,#9644,#9645);
#7740=AXIS2_PLACEMENT_3D('',#12897,#9649,#9650);
#7741=AXIS2_PLACEMENT_3D('',#12899,#9651,#9652);
#7742=AXIS2_PLACEMENT_3D('',#12901,#9653,#9654);
#7743=AXIS2_PLACEMENT_3D('',#12907,#9658,#9659);
#7744=AXIS2_PLACEMENT_3D('',#12909,#9661,#9662);
#7745=AXIS2_PLACEMENT_3D('',#12911,#9663,#9664);
#7746=AXIS2_PLACEMENT_3D('',#12917,#9668,#9669);
#7747=AXIS2_PLACEMENT_3D('',#12922,#9671,#9672);
#7748=AXIS2_PLACEMENT_3D('',#12928,#9676,#9677);
#7749=AXIS2_PLACEMENT_3D('',#12929,#9678,#9679);
#7750=AXIS2_PLACEMENT_3D('',#12933,#9682,#9683);
#7751=AXIS2_PLACEMENT_3D('',#12936,#9685,#9686);
#7752=AXIS2_PLACEMENT_3D('',#12938,#9687,#9688);
#7753=AXIS2_PLACEMENT_3D('',#12941,#9691,#9692);
#7754=AXIS2_PLACEMENT_3D('',#12942,#9693,#9694);
#7755=AXIS2_PLACEMENT_3D('',#12950,#9700,#9701);
#7756=AXIS2_PLACEMENT_3D('',#12957,#9706,#9707);
#7757=AXIS2_PLACEMENT_3D('',#12963,#9711,#9712);
#7758=AXIS2_PLACEMENT_3D('',#12965,#9714,#9715);
#7759=AXIS2_PLACEMENT_3D('',#12966,#9716,#9717);
#7760=AXIS2_PLACEMENT_3D('',#12967,#9718,#9719);
#7761=AXIS2_PLACEMENT_3D('',#12968,#9720,#9721);
#7762=AXIS2_PLACEMENT_3D('',#12969,#9722,#9723);
#7763=AXIS2_PLACEMENT_3D('',#12970,#9724,#9725);
#7764=AXIS2_PLACEMENT_3D('',#12971,#9726,#9727);
#7765=AXIS2_PLACEMENT_3D('',#12972,#9728,#9729);
#7766=AXIS2_PLACEMENT_3D('',#12973,#9730,#9731);
#7767=AXIS2_PLACEMENT_3D('',#12974,#9732,#9733);
#7768=AXIS2_PLACEMENT_3D('',#12975,#9734,#9735);
#7769=AXIS2_PLACEMENT_3D('',#12976,#9736,#9737);
#7770=AXIS2_PLACEMENT_3D('',#12977,#9738,#9739);
#7771=AXIS2_PLACEMENT_3D('',#12978,#9740,#9741);
#7772=AXIS2_PLACEMENT_3D('',#12982,#9745,#9746);
#7773=AXIS2_PLACEMENT_3D('',#12984,#9748,#9749);
#7774=AXIS2_PLACEMENT_3D('',#12985,#9750,#9751);
#7775=AXIS2_PLACEMENT_3D('',#12986,#9752,#9753);
#9543=DIRECTION('axis',(0.,0.,1.));
#9544=DIRECTION('refdir',(1.,0.,0.));
#9545=DIRECTION('center_axis',(0.,-1.,0.));
#9546=DIRECTION('ref_axis',(0.,0.,-1.));
#9547=DIRECTION('center_axis',(0.,-1.,-1.24352412568707E-16));
#9548=DIRECTION('ref_axis',(0.,-1.24352412568707E-16,1.));
#9549=DIRECTION('',(0.,-1.,0.));
#9550=DIRECTION('center_axis',(0.,-1.,0.));
#9551=DIRECTION('ref_axis',(0.,0.,-1.));
#9552=DIRECTION('',(0.,-1.,0.));
#9553=DIRECTION('center_axis',(0.,1.,1.24352412568707E-16));
#9554=DIRECTION('ref_axis',(0.,1.24352412568707E-16,-1.));
#9555=DIRECTION('center_axis',(0.,0.,1.));
#9556=DIRECTION('ref_axis',(1.,0.,0.));
#9557=DIRECTION('center_axis',(0.707106781186583,-1.70853935691577E-13,
0.707106781186512));
#9558=DIRECTION('ref_axis',(0.707106781186512,6.44889800824306E-12,-0.707106781186583));
#9559=DIRECTION('',(0.,0.,1.));
#9560=DIRECTION('center_axis',(-0.707106781186548,0.,0.707106781186548));
#9561=DIRECTION('ref_axis',(0.707106781186547,1.23820750287472E-15,0.707106781186547));
#9562=DIRECTION('',(0.,0.,1.));
#9563=DIRECTION('center_axis',(0.707106781186548,1.36062155274961E-15,-0.707106781186547));
#9564=DIRECTION('ref_axis',(0.707106781186547,-2.36260576158627E-15,0.707106781186548));
#9565=DIRECTION('',(0.,0.,1.));
#9566=DIRECTION('center_axis',(-0.707106781186548,-2.19777105329554E-14,
0.707106781186548));
#9567=DIRECTION('ref_axis',(0.707106781186547,-2.12231778358904E-14,0.707106781186547));
#9568=DIRECTION('',(0.,0.,-1.));
#9569=DIRECTION('center_axis',(0.707106781186576,1.41564689573016E-13,0.707106781186519));
#9570=DIRECTION('ref_axis',(0.707106781186519,3.06847407347585E-11,-0.707106781186576));
#9571=DIRECTION('center_axis',(0.,1.,0.));
#9572=DIRECTION('ref_axis',(0.,0.,1.));
#9573=DIRECTION('center_axis',(0.,-1.,0.));
#9574=DIRECTION('ref_axis',(0.,0.,-1.));
#9575=DIRECTION('',(0.,-1.,0.));
#9576=DIRECTION('center_axis',(0.,1.,0.));
#9577=DIRECTION('ref_axis',(0.,0.,-1.));
#9578=DIRECTION('center_axis',(0.,1.,0.));
#9579=DIRECTION('ref_axis',(0.,0.,1.));
#9580=DIRECTION('center_axis',(0.,-1.,0.));
#9581=DIRECTION('ref_axis',(0.,0.,1.));
#9582=DIRECTION('',(0.,-1.,0.));
#9583=DIRECTION('center_axis',(0.,-1.,0.));
#9584=DIRECTION('ref_axis',(0.,0.,-1.));
#9585=DIRECTION('center_axis',(0.,1.,0.));
#9586=DIRECTION('ref_axis',(0.,0.,1.));
#9587=DIRECTION('center_axis',(0.,-1.,0.));
#9588=DIRECTION('ref_axis',(0.,0.,1.));
#9589=DIRECTION('',(0.,-1.,0.));
#9590=DIRECTION('center_axis',(0.,1.,0.));
#9591=DIRECTION('ref_axis',(0.,0.,-1.));
#9592=DIRECTION('center_axis',(0.,0.,-1.));
#9593=DIRECTION('ref_axis',(-1.,1.20980294963545E-15,0.));
#9594=DIRECTION('center_axis',(0.,0.,1.));
#9595=DIRECTION('ref_axis',(1.,0.,0.));
#9596=DIRECTION('center_axis',(0.,0.,1.));
#9597=DIRECTION('ref_axis',(-1.,0.,0.));
#9598=DIRECTION('center_axis',(0.707106781186548,0.,0.707106781186548));
#9599=DIRECTION('ref_axis',(0.707106781186548,0.,-0.707106781186548));
#9600=DIRECTION('',(-0.707106781186547,0.,0.707106781186547));
#9601=DIRECTION('',(0.,-1.,0.));
#9602=DIRECTION('center_axis',(0.,-1.,0.));
#9603=DIRECTION('ref_axis',(0.,0.,-1.));
#9604=DIRECTION('',(0.707106781186548,0.,0.707106781186548));
#9605=DIRECTION('center_axis',(0.,-1.,0.));
#9606=DIRECTION('ref_axis',(0.,0.,-1.));
#9607=DIRECTION('center_axis',(0.,1.,0.));
#9608=DIRECTION('ref_axis',(0.,0.,1.));
#9609=DIRECTION('',(-0.707106781186547,0.,0.707106781186547));
#9610=DIRECTION('',(-0.707106781186548,0.,-0.707106781186548));
#9611=DIRECTION('center_axis',(0.,1.,0.));
#9612=DIRECTION('ref_axis',(0.,0.,1.));
#9613=DIRECTION('center_axis',(-0.707106781186548,0.,-0.707106781186548));
#9614=DIRECTION('ref_axis',(-0.707106781186548,0.,0.707106781186548));
#9615=DIRECTION('',(-0.707106781186547,0.,0.707106781186547));
#9616=DIRECTION('',(0.,1.,0.));
#9617=DIRECTION('',(-0.707106781186547,0.,0.707106781186547));
#9618=DIRECTION('',(0.,-1.,0.));
#9619=DIRECTION('center_axis',(0.,0.,-1.));
#9620=DIRECTION('ref_axis',(-1.,3.21624529935327E-16,0.));
#9621=DIRECTION('center_axis',(0.,0.,-1.));
#9622=DIRECTION('ref_axis',(1.,1.77635589572802E-15,0.));
#9623=DIRECTION('center_axis',(0.,-1.,0.));
#9624=DIRECTION('ref_axis',(0.,0.,-1.));
#9625=DIRECTION('center_axis',(0.,1.,1.24352412568707E-16));
#9626=DIRECTION('ref_axis',(0.,-1.24352412568707E-16,1.));
#9627=DIRECTION('',(0.,-1.,0.));
#9628=DIRECTION('center_axis',(0.593342281899159,-0.0646221712613811,-0.802352111913568));
#9629=DIRECTION('ref_axis',(-0.738289860535889,-0.440860457545454,-0.510460712300869));
#9630=DIRECTION('',(0.,-1.,0.));
#9631=DIRECTION('center_axis',(0.,-1.,-1.24352412568707E-16));
#9632=DIRECTION('ref_axis',(0.,1.24352412568707E-16,-1.));
#9633=DIRECTION('',(0.,1.,0.));
#9634=DIRECTION('center_axis',(0.999938130553997,0.,0.0111236263950905));
#9635=DIRECTION('ref_axis',(0.0111236263950905,0.,-0.999938130553997));
#9636=DIRECTION('',(0.,-1.,0.));
#9637=DIRECTION('',(0.,1.,0.));
#9638=DIRECTION('center_axis',(0.,0.,1.));
#9639=DIRECTION('ref_axis',(1.,0.,0.));
#9640=DIRECTION('center_axis',(0.,1.,1.24352412568707E-16));
#9641=DIRECTION('ref_axis',(0.,-1.24352412568707E-16,1.));
#9642=DIRECTION('center_axis',(0.,1.,1.24352412568707E-16));
#9643=DIRECTION('ref_axis',(0.,-1.24352412568707E-16,1.));
#9644=DIRECTION('center_axis',(0.,1.,1.24352412568707E-16));
#9645=DIRECTION('ref_axis',(0.,-1.24352412568707E-16,1.));
#9646=DIRECTION('',(0.,1.24352412568707E-16,-1.));
#9647=DIRECTION('',(-1.,0.,0.));
#9648=DIRECTION('',(0.,1.15648231731787E-16,-1.));
#9649=DIRECTION('center_axis',(0.,-1.,-1.24352412568707E-16));
#9650=DIRECTION('ref_axis',(0.,1.24352412568707E-16,-1.));
#9651=DIRECTION('center_axis',(0.,-1.,-1.24352412568707E-16));
#9652=DIRECTION('ref_axis',(0.,1.24352412568707E-16,-1.));
#9653=DIRECTION('center_axis',(0.,-1.,-1.24352412568707E-16));
#9654=DIRECTION('ref_axis',(0.,1.24352412568707E-16,-1.));
#9655=DIRECTION('',(0.,1.15648231731787E-16,-1.));
#9656=DIRECTION('',(1.,-2.15636651137065E-16,0.));
#9657=DIRECTION('',(0.,-1.24352412568707E-16,1.));
#9658=DIRECTION('center_axis',(-1.,0.,0.));
#9659=DIRECTION('ref_axis',(0.,0.,1.));
#9660=DIRECTION('',(0.,1.,2.10269512239613E-16));
#9661=DIRECTION('center_axis',(0.,0.,1.));
#9662=DIRECTION('ref_axis',(1.,0.,0.));
#9663=DIRECTION('center_axis',(0.,0.,-1.));
#9664=DIRECTION('ref_axis',(1.,0.,0.));
#9665=DIRECTION('',(-1.,0.,0.));
#9666=DIRECTION('',(0.,1.,0.));
#9667=DIRECTION('',(-1.,0.,0.));
#9668=DIRECTION('center_axis',(0.,-1.,0.));
#9669=DIRECTION('ref_axis',(0.,0.,-1.));
#9670=DIRECTION('',(0.707106781186547,0.,-0.707106781186547));
#9671=DIRECTION('center_axis',(0.,1.,0.));
#9672=DIRECTION('ref_axis',(0.,0.,-1.));
#9673=DIRECTION('',(0.707106781186548,0.,0.707106781186548));
#9674=DIRECTION('',(-1.,0.,0.));
#9675=DIRECTION('',(0.707106781186548,0.,0.707106781186548));
#9676=DIRECTION('center_axis',(0.,1.,0.));
#9677=DIRECTION('ref_axis',(3.15404268359419E-15,0.,-1.));
#9678=DIRECTION('center_axis',(0.,0.,-1.));
#9679=DIRECTION('ref_axis',(-1.,0.,0.));
#9680=DIRECTION('',(0.,-1.,0.));
#9681=DIRECTION('',(-1.,0.,0.));
#9682=DIRECTION('center_axis',(0.,1.,0.));
#9683=DIRECTION('ref_axis',(0.,0.,1.));
#9684=DIRECTION('',(0.707106781186548,0.,0.707106781186548));
#9685=DIRECTION('center_axis',(0.,-1.,0.));
#9686=DIRECTION('ref_axis',(3.15404268359419E-15,0.,1.));
#9687=DIRECTION('center_axis',(0.,-1.,0.));
#9688=DIRECTION('ref_axis',(-3.15404268359419E-15,0.,1.));
#9689=DIRECTION('',(0.707106781186548,0.,0.707106781186548));
#9690=DIRECTION('',(-0.0186217163628307,0.,-0.999826600806211));
#9691=DIRECTION('center_axis',(0.,0.,-1.));
#9692=DIRECTION('ref_axis',(1.,0.,0.));
#9693=DIRECTION('center_axis',(-0.707106781186548,0.,0.707106781186547));
#9694=DIRECTION('ref_axis',(0.707106781186547,0.,0.707106781186548));
#9695=DIRECTION('',(-0.707106781186548,0.,-0.707106781186548));
#9696=DIRECTION('',(0.,1.,0.));
#9697=DIRECTION('',(0.,1.,0.));
#9698=DIRECTION('',(0.707106781186548,0.,0.707106781186548));
#9699=DIRECTION('',(0.,1.,0.));
#9700=DIRECTION('center_axis',(0.707106781186548,0.,-0.707106781186547));
#9701=DIRECTION('ref_axis',(-0.707106781186547,0.,-0.707106781186548));
#9702=DIRECTION('',(-0.707106781186548,0.,-0.707106781186548));
#9703=DIRECTION('',(0.707106781186548,0.,0.707106781186548));
#9704=DIRECTION('',(0.,-1.,0.));
#9705=DIRECTION('',(0.,-1.,0.));
#9706=DIRECTION('center_axis',(-0.707106781186548,0.,-0.707106781186548));
#9707=DIRECTION('ref_axis',(-0.707106781186548,0.,0.707106781186548));
#9708=DIRECTION('',(0.707106781186547,0.,-0.707106781186547));
#9709=DIRECTION('',(0.,1.,0.));
#9710=DIRECTION('',(0.,-1.,0.));
#9711=DIRECTION('center_axis',(0.707106781186548,0.,0.707106781186548));
#9712=DIRECTION('ref_axis',(0.707106781186548,0.,-0.707106781186548));
#9713=DIRECTION('',(0.,-1.,0.));
#9714=DIRECTION('center_axis',(0.,-1.,0.));
#9715=DIRECTION('ref_axis',(0.,0.,-1.));
#9716=DIRECTION('center_axis',(0.,1.,0.));
#9717=DIRECTION('ref_axis',(-6.30808536718839E-15,0.,-1.));
#9718=DIRECTION('center_axis',(0.,1.,0.));
#9719=DIRECTION('ref_axis',(-3.1540426835942E-15,0.,-1.));
#9720=DIRECTION('center_axis',(0.,1.,0.));
#9721=DIRECTION('ref_axis',(0.,0.,1.));
#9722=DIRECTION('center_axis',(0.,-1.,0.));
#9723=DIRECTION('ref_axis',(0.,0.,1.));
#9724=DIRECTION('center_axis',(0.,-1.,0.));
#9725=DIRECTION('ref_axis',(-3.15404268359419E-15,0.,1.));
#9726=DIRECTION('center_axis',(0.,-1.,0.));
#9727=DIRECTION('ref_axis',(0.,0.,-1.));
#9728=DIRECTION('center_axis',(0.,-1.,0.));
#9729=DIRECTION('ref_axis',(0.,0.,-1.));
#9730=DIRECTION('center_axis',(0.,-1.,0.));
#9731=DIRECTION('ref_axis',(0.,0.,-1.));
#9732=DIRECTION('center_axis',(0.,-1.,0.));
#9733=DIRECTION('ref_axis',(0.,0.,-1.));
#9734=DIRECTION('center_axis',(0.,1.,0.));
#9735=DIRECTION('ref_axis',(2.78699993901511E-15,0.,-1.));
#9736=DIRECTION('center_axis',(0.,1.,0.));
#9737=DIRECTION('ref_axis',(2.78699993901511E-15,0.,-1.));
#9738=DIRECTION('center_axis',(0.,1.,0.));
#9739=DIRECTION('ref_axis',(-1.89882151931499E-15,0.,-1.));
#9740=DIRECTION('center_axis',(0.,1.,0.));
#9741=DIRECTION('ref_axis',(0.,0.,1.));
#9742=DIRECTION('',(0.,1.,0.));
#9743=DIRECTION('',(0.,1.,0.));
#9744=DIRECTION('',(0.,1.,0.));
#9745=DIRECTION('center_axis',(1.,0.,0.));
#9746=DIRECTION('ref_axis',(0.,0.,-1.));
#9747=DIRECTION('',(0.,-1.,-2.10269512239613E-16));
#9748=DIRECTION('center_axis',(4.53418134555742E-32,2.10269512239613E-16,
-1.));
#9749=DIRECTION('ref_axis',(0.,1.,2.10269512239613E-16));
#9750=DIRECTION('center_axis',(0.,1.,0.));
#9751=DIRECTION('ref_axis',(0.,0.,1.));
#9752=DIRECTION('center_axis',(0.,1.,0.));
#9753=DIRECTION('ref_axis',(0.,0.,1.));
#12588=CARTESIAN_POINT('',(0.,0.,0.));
#12589=CARTESIAN_POINT('Origin',(0.110247934021453,18.,10.8869317850633));
#12590=CARTESIAN_POINT('',(0.110247934021453,-8.24965010070131,12.3869317850633));
#12591=CARTESIAN_POINT('Origin',(0.110247934021453,-8.24965010070131,10.8869317850633));
#12592=CARTESIAN_POINT('',(0.110247933887646,-14.0552557433871,12.3869317850633));
#12593=CARTESIAN_POINT('',(0.110247934021453,18.,12.3869317850633));
#12594=CARTESIAN_POINT('',(0.110247934021453,-14.1076210252064,9.3869317850633));
#12595=CARTESIAN_POINT('Ctrl Pts',(0.110247933753838,-14.0552557433871,
12.3869317850633));
#12596=CARTESIAN_POINT('Ctrl Pts',(-0.0779989827009714,-14.0549118893516,
12.3869317850297));
#12597=CARTESIAN_POINT('Ctrl Pts',(-0.278728344791251,-14.0510324275907,
12.3493319245718));
#12598=CARTESIAN_POINT('Ctrl Pts',(-0.647959467681628,-14.0379478709213,
12.1965290487721));
#12599=CARTESIAN_POINT('Ctrl Pts',(-0.816468494212286,-14.0289559136302,
12.0813250316921));
#12600=CARTESIAN_POINT('Ctrl Pts',(-1.08260740435852,-14.0130041171202,
11.8156060213132));
#12601=CARTESIAN_POINT('Ctrl Pts',(-1.19805838607211,-14.0050121842533,
11.6473460303996));
#12602=CARTESIAN_POINT('Ctrl Pts',(-1.3514541799802,-13.9960274725997,11.2784955234755));
#12603=CARTESIAN_POINT('Ctrl Pts',(-1.38939360404563,-13.9952553156971,
11.0778974256665));
#12604=CARTESIAN_POINT('Ctrl Pts',(-1.39010647607766,-14.0017963063311,
10.7009453898944));
#12605=CARTESIAN_POINT('Ctrl Pts',(-1.35266265154803,-14.0095718793367,
10.4996613198593));
#12606=CARTESIAN_POINT('Ctrl Pts',(-1.19987566293113,-14.0314540986523,
10.1295270026253));
#12607=CARTESIAN_POINT('Ctrl Pts',(-1.08454283481342,-14.0453388880625,
9.96065940627607));
#12608=CARTESIAN_POINT('Ctrl Pts',(-0.818352054767195,-14.0705968835703,
9.69395625658189));
#12609=CARTESIAN_POINT('Ctrl Pts',(-0.649705142487691,-14.0836248485775,
9.5782824456212));
#12610=CARTESIAN_POINT('Ctrl Pts',(-0.279839795725651,-14.1020716632627,
9.42476786050772));
#12611=CARTESIAN_POINT('Ctrl Pts',(-0.078606279092388,-14.1072765984644,
9.38693779445533));
#12612=CARTESIAN_POINT('Ctrl Pts',(0.110216109641043,-14.1076209672601,
9.3869317853165));
#12613=CARTESIAN_POINT('Ctrl Pts',(0.110232021787044,-14.1076209962489,
9.3869317850633));
#12614=CARTESIAN_POINT('Ctrl Pts',(0.110247934021453,-14.1076210252064,
9.3869317850633));
#12615=CARTESIAN_POINT('Ctrl Pts',(0.110247934021453,-14.1076210252064,
9.3869317850633));
#12616=CARTESIAN_POINT('Ctrl Pts',(0.299018164756681,-14.1079645552822,
9.3869317850633));
#12617=CARTESIAN_POINT('Ctrl Pts',(0.500231125056626,-14.1034945808851,
9.42474185766269));
#12618=CARTESIAN_POINT('Ctrl Pts',(0.870098969070737,-14.0864013169578,
9.57822271524134));
#12619=CARTESIAN_POINT('Ctrl Pts',(1.03876516505625,-14.0739913371949,9.69389031798828));
#12620=CARTESIAN_POINT('Ctrl Pts',(1.30499104641839,-14.0497109843586,9.96059468363198));
#12621=CARTESIAN_POINT('Ctrl Pts',(1.42033561388508,-14.0362517791226,10.1294648498598));
#12622=CARTESIAN_POINT('Ctrl Pts',(1.57314021718156,-14.0149355408367,10.4995921319432));
#12623=CARTESIAN_POINT('Ctrl Pts',(1.61059047387225,-14.0072999254605,10.700866003491));
#12624=CARTESIAN_POINT('Ctrl Pts',(1.61024542921315,-14.0040223989729,10.8896730290548));
#12625=CARTESIAN_POINT('Ctrl Pts',(1.60990162279029,-14.000756634302,11.0778024968157));
#12626=CARTESIAN_POINT('Ctrl Pts',(1.57197504847848,-14.0013878345693,11.2784068501416));
#12627=CARTESIAN_POINT('Ctrl Pts',(1.41859248113633,-14.0098055316953,11.6472826572499));
#12628=CARTESIAN_POINT('Ctrl Pts',(1.30314144421112,-14.0173717863179,11.8155611648083));
#12629=CARTESIAN_POINT('Ctrl Pts',(1.03699817477234,-14.032345318826,12.0812980188678));
#12630=CARTESIAN_POINT('Ctrl Pts',(0.868493391579155,-14.0407189153297,
12.196505971612));
#12631=CARTESIAN_POINT('Ctrl Pts',(0.499264482529693,-14.052452711895,12.3493225855658));
#12632=CARTESIAN_POINT('Ctrl Pts',(0.298531336987817,-14.0555991292645,
12.3869257938369));
#12633=CARTESIAN_POINT('Ctrl Pts',(0.110279758313445,-14.0552558014956,
12.3869317848101));
#12634=CARTESIAN_POINT('Ctrl Pts',(0.110263846078239,-14.0552557724528,
12.3869317850633));
#12635=CARTESIAN_POINT('Ctrl Pts',(0.110247933753838,-14.0552557433871,
12.3869317850633));
#12636=CARTESIAN_POINT('Origin',(0.110247934021453,18.,10.8869317850633));
#12637=CARTESIAN_POINT('',(0.110247934021807,14.1083208238043,9.38693178505972));
#12638=CARTESIAN_POINT('',(0.110247933887645,14.0559555419845,12.3869317850633));
#12639=CARTESIAN_POINT('Ctrl Pts',(0.110247934021808,14.1083208238038,9.3869317850633));
#12640=CARTESIAN_POINT('Ctrl Pts',(0.110232021787281,14.1083207948462,9.3869317850633));
#12641=CARTESIAN_POINT('Ctrl Pts',(0.11021610964116,14.1083207658575,9.3869317853165));
#12642=CARTESIAN_POINT('Ctrl Pts',(-0.0786062790923889,14.1079763970618,
9.38693779445533));
#12643=CARTESIAN_POINT('Ctrl Pts',(-0.279839795725652,14.1027714618601,
9.42476786050772));
#12644=CARTESIAN_POINT('Ctrl Pts',(-0.649705142487692,14.0843246471749,
9.57828244562119));
#12645=CARTESIAN_POINT('Ctrl Pts',(-0.818352054767195,14.0712966821677,
9.69395625658189));
#12646=CARTESIAN_POINT('Ctrl Pts',(-1.08454283481342,14.0460386866599,9.96065940627607));
#12647=CARTESIAN_POINT('Ctrl Pts',(-1.19987566293113,14.0321538972497,10.1295270026253));
#12648=CARTESIAN_POINT('Ctrl Pts',(-1.35266265154803,14.0102716779341,10.4996613198593));
#12649=CARTESIAN_POINT('Ctrl Pts',(-1.39010647607766,14.0024961049285,10.7009453898944));
#12650=CARTESIAN_POINT('Ctrl Pts',(-1.38939360404563,13.9959551142944,11.0778974256665));
#12651=CARTESIAN_POINT('Ctrl Pts',(-1.3514541799802,13.9967272711971,11.2784955234755));
#12652=CARTESIAN_POINT('Ctrl Pts',(-1.19805838607211,14.0057119828507,11.6473460303996));
#12653=CARTESIAN_POINT('Ctrl Pts',(-1.08260740435852,14.0137039157176,11.8156060213132));
#12654=CARTESIAN_POINT('Ctrl Pts',(-0.816468494212286,14.0296557122276,
12.0813250316921));
#12655=CARTESIAN_POINT('Ctrl Pts',(-0.647959467681628,14.0386476695187,
12.1965290487721));
#12656=CARTESIAN_POINT('Ctrl Pts',(-0.278728344791252,14.051732226188,12.3493319245718));
#12657=CARTESIAN_POINT('Ctrl Pts',(-0.0779989827009722,14.055611687949,
12.3869317850297));
#12658=CARTESIAN_POINT('Ctrl Pts',(0.110247933753837,14.0559555419845,12.3869317850633));
#12659=CARTESIAN_POINT('',(0.110247934021453,8.25034989929869,12.3869317850633));
#12660=CARTESIAN_POINT('',(0.110247934021453,18.,12.3869317850633));
#12661=CARTESIAN_POINT('Origin',(0.110247934021453,8.25034989929869,10.8869317850633));
#12662=CARTESIAN_POINT('Ctrl Pts',(0.110247933753837,14.0559555419845,12.3869317850633));
#12663=CARTESIAN_POINT('Ctrl Pts',(0.110263846078238,14.0559555710501,12.3869317850633));
#12664=CARTESIAN_POINT('Ctrl Pts',(0.110279758313445,14.055955600093,12.3869317848101));
#12665=CARTESIAN_POINT('Ctrl Pts',(0.298531336987817,14.0562989278619,12.3869257938369));
#12666=CARTESIAN_POINT('Ctrl Pts',(0.499264482529694,14.0531525104924,12.3493225855658));
#12667=CARTESIAN_POINT('Ctrl Pts',(0.868493391579156,14.0414187139271,12.196505971612));
#12668=CARTESIAN_POINT('Ctrl Pts',(1.03699817477234,14.0330451174234,12.0812980188678));
#12669=CARTESIAN_POINT('Ctrl Pts',(1.30314144421112,14.0180715849152,11.8155611648083));
#12670=CARTESIAN_POINT('Ctrl Pts',(1.41859248113633,14.0105053302927,11.6472826572499));
#12671=CARTESIAN_POINT('Ctrl Pts',(1.57197504847848,14.0020876331667,11.2784068501416));
#12672=CARTESIAN_POINT('Ctrl Pts',(1.60990162279029,14.0014564328994,11.0778024968157));
#12673=CARTESIAN_POINT('Ctrl Pts',(1.61024542921315,14.0047221975703,10.8896730290548));
#12674=CARTESIAN_POINT('Ctrl Pts',(1.61059047387225,14.0079997240579,10.700866003491));
#12675=CARTESIAN_POINT('Ctrl Pts',(1.57314021718156,14.0156353394341,10.4995921319432));
#12676=CARTESIAN_POINT('Ctrl Pts',(1.42033561388508,14.03695157772,10.1294648498598));
#12677=CARTESIAN_POINT('Ctrl Pts',(1.30499104641839,14.050410782956,9.96059468363198));
#12678=CARTESIAN_POINT('Ctrl Pts',(1.03876516505625,14.0746911357923,9.69389031798828));
#12679=CARTESIAN_POINT('Ctrl Pts',(0.870098969070735,14.0871011155552,9.57822271524134));
#12680=CARTESIAN_POINT('Ctrl Pts',(0.500231125056741,14.1041943794824,9.42474185766273));
#12681=CARTESIAN_POINT('Ctrl Pts',(0.299018164756932,14.1086643538796,9.38693178506334));
#12682=CARTESIAN_POINT('Ctrl Pts',(0.110247934021808,14.1083208238038,9.3869317850633));
#12683=CARTESIAN_POINT('Origin',(-17.8485597402224,-0.120323143610449,-16.1677081946201));
#12684=CARTESIAN_POINT('',(-16.497528189245,2.37951225022575,-1.54552565392526));
#12685=CARTESIAN_POINT('',(-16.497528189245,-2.62015853744665,-1.54552565392526));
#12686=CARTESIAN_POINT('Ctrl Pts',(-16.4975281892429,2.37951225022459,-1.54552565392739));
#12687=CARTESIAN_POINT('Ctrl Pts',(-16.420741563328,2.33801305609358,-1.62231227984189));
#12688=CARTESIAN_POINT('Ctrl Pts',(-16.3240357866784,2.27985744112584,-1.69185037854978));
#12689=CARTESIAN_POINT('Ctrl Pts',(-16.0647935003745,2.10171647680498,-1.83077158616984));
#12690=CARTESIAN_POINT('Ctrl Pts',(-15.8578857100574,1.92056821996525,-1.86953234897271));
#12691=CARTESIAN_POINT('Ctrl Pts',(-15.4883556328401,1.49633440199585,-1.86488639419025));
#12692=CARTESIAN_POINT('Ctrl Pts',(-15.3080382336862,1.19791710112843,-1.79698849462938));
#12693=CARTESIAN_POINT('Ctrl Pts',(-15.0674088041674,0.555842639994981,
-1.66403388485253));
#12694=CARTESIAN_POINT('Ctrl Pts',(-15.0069997376864,0.210870575808918,
-1.60558828241371));
#12695=CARTESIAN_POINT('Ctrl Pts',(-15.0069997376864,-0.451516863029818,
-1.60558828241371));
#12696=CARTESIAN_POINT('Ctrl Pts',(-15.0674088041674,-0.79648892721588,
-1.66403388485253));
#12697=CARTESIAN_POINT('Ctrl Pts',(-15.3080382336862,-1.43856338834933,
-1.79698849462938));
#12698=CARTESIAN_POINT('Ctrl Pts',(-15.4883556328401,-1.73698068921675,
-1.86488639419025));
#12699=CARTESIAN_POINT('Ctrl Pts',(-15.8578857100574,-2.16121450718615,
-1.86953234897271));
#12700=CARTESIAN_POINT('Ctrl Pts',(-16.0647935003745,-2.34236276402588,
-1.83077158616984));
#12701=CARTESIAN_POINT('Ctrl Pts',(-16.3240357866792,-2.52050372834728,
-1.69185037854936));
#12702=CARTESIAN_POINT('Ctrl Pts',(-16.4207415633297,-2.57865934331552,
-1.62231227984055));
#12703=CARTESIAN_POINT('Ctrl Pts',(-16.497528189245,-2.62015853744664,-1.54552565392525));
#12704=CARTESIAN_POINT('',(-17.1330436691154,-2.87032314361045,-0.910010174054937));
#12705=CARTESIAN_POINT('Origin',(-17.8485597402078,-0.120323143639212,-0.194494102961751));
#12706=CARTESIAN_POINT('',(-17.1330436691154,-2.87032314361045,-3.73667605240598));
#12707=CARTESIAN_POINT('',(-17.1330436691154,-2.87032314361045,-16.1677081946201));
#12708=CARTESIAN_POINT('',(-18.5640758113294,-2.87032314361045,-5.16770819462005));
#12709=CARTESIAN_POINT('Origin',(-17.8485597402224,-0.120323143607889,-4.45219212351302));
#12710=CARTESIAN_POINT('',(-18.5640758113294,-2.87032314361045,1.43229180537995));
#12711=CARTESIAN_POINT('',(-18.5640758113294,-2.87032314361045,-16.1677081946201));
#12712=CARTESIAN_POINT('',(-18.5640758113294,2.62967685638955,1.43229180537995));
#12713=CARTESIAN_POINT('Origin',(-17.8485597402224,-0.120323143610436,2.14780787648699));
#12714=CARTESIAN_POINT('',(-18.5640758113294,2.62967685638955,-5.16770819462005));
#12715=CARTESIAN_POINT('',(-18.5640758113294,2.62967685638955,-16.1677081946201));
#12716=CARTESIAN_POINT('',(-17.1330436691154,2.62967685638955,-3.73667605240598));
#12717=CARTESIAN_POINT('Origin',(-17.8485597402223,-0.120323143614262,-4.45219212351302));
#12718=CARTESIAN_POINT('',(-17.1330436691154,2.62967685638955,-0.910010174054937));
#12719=CARTESIAN_POINT('',(-17.1330436691154,2.62967685638955,-16.1677081946201));
#12720=CARTESIAN_POINT('Origin',(-17.8485597402879,-0.120323143780666,-0.194494102881747));
#12721=CARTESIAN_POINT('Origin',(-19.7031631078554,-6.08245867427902,-3.00679549114607));
#12722=CARTESIAN_POINT('',(-19.7031631078554,5.84154132572098,-4.10679549114607));
#12723=CARTESIAN_POINT('Origin',(-19.7031631078554,5.84154132572098,-3.00679549114607));
#12724=CARTESIAN_POINT('',(-19.7031631078554,4.74181238705812,-4.10679549114607));
#12725=CARTESIAN_POINT('',(-19.7031631078554,-6.08245867427902,-4.10679549114607));
#12726=CARTESIAN_POINT('Origin',(-19.7031631078554,4.74181238705812,-3.00679549114607));
#12727=CARTESIAN_POINT('Origin',(-19.7031631078554,-6.08245867427902,-3.00679549114607));
#12728=CARTESIAN_POINT('',(-19.7031631078554,-4.98245867427902,-4.10679549114607));
#12729=CARTESIAN_POINT('Origin',(-19.7031631078554,-4.98245867427902,-3.00679549114607));
#12730=CARTESIAN_POINT('',(-19.7031631078554,-6.08245867427902,-4.10679549114607));
#12731=CARTESIAN_POINT('',(-19.7031631078554,-6.08245867427902,-4.10679549114607));
#12732=CARTESIAN_POINT('Origin',(-19.7031631078554,-6.08245867427902,-3.00679549114607));
#12733=CARTESIAN_POINT('Origin',(-19.7031631078554,-6.08245867427902,-3.00679549114607));
#12734=CARTESIAN_POINT('',(-19.7031631078554,2.62967685638955,-4.10679549114607));
#12735=CARTESIAN_POINT('Origin',(-19.7031631078554,2.62967685638955,-3.00679549114607));
#12736=CARTESIAN_POINT('',(-19.7031631078554,-2.87032314361045,-4.10679549114607));
#12737=CARTESIAN_POINT('',(-19.7031631078554,-6.08245867427902,-4.10679549114607));
#12738=CARTESIAN_POINT('Origin',(-19.7031631078554,-2.87032314361045,-3.00679549114607));
#12739=CARTESIAN_POINT('Origin',(0.135922068665986,0.000349899298694283,
-1.61306821493671));
#12740=CARTESIAN_POINT('',(-5.08045717850762,-13.2101970980443,3.93608070944324));
#12741=CARTESIAN_POINT('',(-13.2505381529841,-4.98245867427902,-0.68247630754827));
#12742=CARTESIAN_POINT('Ctrl Pts',(-5.08045717850762,-13.2101970980444,
3.93608070944324));
#12743=CARTESIAN_POINT('Ctrl Pts',(-5.19427083564475,-13.1658432312101,
3.90479457078127));
#12744=CARTESIAN_POINT('Ctrl Pts',(-5.30737084438806,-13.1200941149079,
3.87257838053821));
#12745=CARTESIAN_POINT('Ctrl Pts',(-7.16749797466,-12.340014395333,3.32439961684679));
#12746=CARTESIAN_POINT('Ctrl Pts',(-8.72366651892778,-11.2620710679717,
2.58238150810523));
#12747=CARTESIAN_POINT('Ctrl Pts',(-11.1912637350643,-8.82660940607619,
1.08947071342651));
#12748=CARTESIAN_POINT('Ctrl Pts',(-12.2765811993519,-7.2824004800094,0.21805432518995));
#12749=CARTESIAN_POINT('Ctrl Pts',(-13.1000234307682,-5.36685264522708,
-0.540299360151207));
#12750=CARTESIAN_POINT('Ctrl Pts',(-13.1773264791433,-5.17565684815307,
-0.612785264279329));
#12751=CARTESIAN_POINT('Ctrl Pts',(-13.2505381529841,-4.98245867427907,
-0.682476307548427));
#12752=CARTESIAN_POINT('',(-0.117610192876321,-14.14538010659,7.09490065582709));
#12753=CARTESIAN_POINT('Ctrl Pts',(-5.08045717850762,-13.2101970980444,
3.93608070944324));
#12754=CARTESIAN_POINT('Ctrl Pts',(-4.64036715107621,-13.3817028291032,
4.05705667988745));
#12755=CARTESIAN_POINT('Ctrl Pts',(-4.20677536912925,-13.5243909716407,
4.20923394033941));
#12756=CARTESIAN_POINT('Ctrl Pts',(-3.28371616224739,-13.7831397146222,
4.60459023494974));
#12757=CARTESIAN_POINT('Ctrl Pts',(-2.73813134372595,-13.9017566032157,
4.8919833150883));
#12758=CARTESIAN_POINT('Ctrl Pts',(-1.70519120635403,-14.0638413625729,
5.57389167932221));
#12759=CARTESIAN_POINT('Ctrl Pts',(-1.21811780812576,-14.1085223634017,
5.96854508266688));
#12760=CARTESIAN_POINT('Ctrl Pts',(-0.56724899223391,-14.1409328592556,
6.59350219068028));
#12761=CARTESIAN_POINT('Ctrl Pts',(-0.33704980837108,-14.1459457009925,
6.83721828261811));
#12762=CARTESIAN_POINT('Ctrl Pts',(-0.117610192876322,-14.14538010659,7.09490065582709));
#12763=CARTESIAN_POINT('',(13.9997902889911,-1.74673802437828,17.0911694938297));
#12764=CARTESIAN_POINT('Ctrl Pts',(-0.117610192876319,-14.14538010659,7.09490065582709));
#12765=CARTESIAN_POINT('Ctrl Pts',(0.287626138302845,-14.1443356306413,
7.57075939853091));
#12766=CARTESIAN_POINT('Ctrl Pts',(0.703875256497269,-14.1263201117739,
8.03375426636872));
#12767=CARTESIAN_POINT('Ctrl Pts',(2.81839943242586,-13.9381054957977,10.2645152922982));
#12768=CARTESIAN_POINT('Ctrl Pts',(4.66337005253943,-13.4890535959015,11.8309862161255));
#12769=CARTESIAN_POINT('Ctrl Pts',(7.56897014261126,-11.9529562948628,13.8505592189385));
#12770=CARTESIAN_POINT('Ctrl Pts',(8.64240851599456,-11.2215374031172,14.5111965660852));
#12771=CARTESIAN_POINT('Ctrl Pts',(10.5894885169921,-9.40644175625714,15.5873518377379));
#12772=CARTESIAN_POINT('Ctrl Pts',(11.4595922188052,-8.32118933554518,16.0066065835401));
#12773=CARTESIAN_POINT('Ctrl Pts',(12.7253532066206,-6.19615494318079,16.5792764506805));
#12774=CARTESIAN_POINT('Ctrl Pts',(13.2509932310767,-5.00707161202048,16.7956436259973));
#12775=CARTESIAN_POINT('Ctrl Pts',(13.7806562363602,-3.09709539960396,17.0067163827827));
#12776=CARTESIAN_POINT('Ctrl Pts',(13.9157062376927,-2.41849085402253,17.058858010685));
#12777=CARTESIAN_POINT('Ctrl Pts',(13.9997902889911,-1.74673802437828,17.0911694938297));
#12778=CARTESIAN_POINT('',(13.9019434616744,-1.21975671714985,25.8869317850633));
#12779=CARTESIAN_POINT('Ctrl Pts',(13.9019434616756,-1.21975671715783,25.8869317849523));
#12780=CARTESIAN_POINT('Ctrl Pts',(13.9421779524689,-1.48088863696913,22.2701255314285));
#12781=CARTESIAN_POINT('Ctrl Pts',(13.9997902889911,-1.74673802437823,17.0911694938297));
#12782=CARTESIAN_POINT('',(13.9019434616744,1.22045651574723,25.8869317850633));
#12783=CARTESIAN_POINT('Origin',(0.135922068665986,0.000349899298694283,
25.8869317850633));
#12784=CARTESIAN_POINT('',(13.9997902889911,1.74743782297565,17.0911694938297));
#12785=CARTESIAN_POINT('Ctrl Pts',(13.9997902889911,1.74743782297562,17.0911694938297));
#12786=CARTESIAN_POINT('Ctrl Pts',(13.942177952468,1.48158843556245,22.2701255315078));
#12787=CARTESIAN_POINT('Ctrl Pts',(13.9019434616744,1.2204565157472,25.8869317850633));
#12788=CARTESIAN_POINT('',(-0.117610192876318,14.1460799051874,7.09490065582708));
#12789=CARTESIAN_POINT('Ctrl Pts',(13.9997902889911,1.74743782297566,17.0911694938297));
#12790=CARTESIAN_POINT('Ctrl Pts',(13.9157062376927,2.41919065261991,17.058858010685));
#12791=CARTESIAN_POINT('Ctrl Pts',(13.7806562363602,3.09779519820135,17.0067163827827));
#12792=CARTESIAN_POINT('Ctrl Pts',(13.2509932310767,5.00777141061787,16.7956436259973));
#12793=CARTESIAN_POINT('Ctrl Pts',(12.7253532066206,6.19685474177818,16.5792764506805));
#12794=CARTESIAN_POINT('Ctrl Pts',(11.4595922188052,8.32188913414257,16.0066065835401));
#12795=CARTESIAN_POINT('Ctrl Pts',(10.5894885169921,9.40714155485452,15.5873518377379));
#12796=CARTESIAN_POINT('Ctrl Pts',(8.64240851599456,11.2222372017146,14.5111965660852));
#12797=CARTESIAN_POINT('Ctrl Pts',(7.56897014261126,11.9536560934602,13.8505592189385));
#12798=CARTESIAN_POINT('Ctrl Pts',(4.66337005253943,13.4897533944989,11.8309862161255));
#12799=CARTESIAN_POINT('Ctrl Pts',(2.81839943242586,13.9388052943951,10.2645152922982));
#12800=CARTESIAN_POINT('Ctrl Pts',(0.703875256497267,14.1270199103713,8.03375426636873));
#12801=CARTESIAN_POINT('Ctrl Pts',(0.287626138302846,14.1450354292387,7.57075939853092));
#12802=CARTESIAN_POINT('Ctrl Pts',(-0.117610192876319,14.1460799051874,
7.09490065582709));
#12803=CARTESIAN_POINT('',(-5.08045717850761,13.2108968966417,3.93608070944324));
#12804=CARTESIAN_POINT('Ctrl Pts',(-0.117610192876326,14.1460799051874,
7.09490065582709));
#12805=CARTESIAN_POINT('Ctrl Pts',(-0.337049808371082,14.1466454995899,
6.83721828261811));
#12806=CARTESIAN_POINT('Ctrl Pts',(-0.56724899223391,14.141632657853,6.59350219068028));
#12807=CARTESIAN_POINT('Ctrl Pts',(-1.21811780812576,14.1092221619991,5.96854508266688));
#12808=CARTESIAN_POINT('Ctrl Pts',(-1.70519120635403,14.0645411611703,5.57389167932221));
#12809=CARTESIAN_POINT('Ctrl Pts',(-2.73813134372595,13.9024564018131,4.8919833150883));
#12810=CARTESIAN_POINT('Ctrl Pts',(-3.28371616224739,13.7838395132195,4.60459023494974));
#12811=CARTESIAN_POINT('Ctrl Pts',(-4.20677536912925,13.5250907702381,4.20923394033941));
#12812=CARTESIAN_POINT('Ctrl Pts',(-4.6403671510762,13.3824026277006,4.05705667988745));
#12813=CARTESIAN_POINT('Ctrl Pts',(-5.0804571785076,13.2108968966417,3.93608070944325));
#12814=CARTESIAN_POINT('',(-13.3394911057634,4.74181001551124,-0.767702265509899));
#12815=CARTESIAN_POINT('Ctrl Pts',(-13.3394914716453,4.74180804892938,-0.76769619274218));
#12816=CARTESIAN_POINT('Ctrl Pts',(-13.2407555507495,5.0174130007776,-0.672496539421838));
#12817=CARTESIAN_POINT('Ctrl Pts',(-13.1337092699761,5.28919013266817,-0.5713225204076));
#12818=CARTESIAN_POINT('Ctrl Pts',(-12.2765811993519,7.28310027860678,0.218054325189944));
#12819=CARTESIAN_POINT('Ctrl Pts',(-11.1912637350643,8.82730920467356,1.08947071342651));
#12820=CARTESIAN_POINT('Ctrl Pts',(-8.72366651892778,11.2627708665691,2.58238150810522));
#12821=CARTESIAN_POINT('Ctrl Pts',(-7.16749797466001,12.3407141939304,3.32439961684678));
#12822=CARTESIAN_POINT('Ctrl Pts',(-5.30737084438806,13.1207939135053,3.87257838053821));
#12823=CARTESIAN_POINT('Ctrl Pts',(-5.19427083564474,13.1665430298075,3.90479457078127));
#12824=CARTESIAN_POINT('Ctrl Pts',(-5.08045717850761,13.2108968966417,3.93608070944324));
#12825=CARTESIAN_POINT('',(-13.2173018321168,4.74181238705812,5.83229180537995));
#12826=CARTESIAN_POINT('Ctrl Pts',(-13.339490057964,4.74181238705812,-0.767702284898452));
#12827=CARTESIAN_POINT('Ctrl Pts',(-13.2781486012827,4.74181238705812,2.54732423788973));
#12828=CARTESIAN_POINT('Ctrl Pts',(-13.2173018321188,4.74181238705812,5.83229180540079));
#12829=CARTESIAN_POINT('',(-13.1291325405826,-4.98245867427902,5.83229180537995));
#12830=CARTESIAN_POINT('Origin',(0.135922068665986,0.000349899298694283,
5.83229180537995));
#12831=CARTESIAN_POINT('Ctrl Pts',(-13.1291325405826,-4.98245867427902,
5.83229180537995));
#12832=CARTESIAN_POINT('Ctrl Pts',(-13.1493356074637,-4.98245867427902,
4.74877968014184));
#12833=CARTESIAN_POINT('Ctrl Pts',(-13.1898154199253,-4.98245867427902,
2.57719051924169));
#12834=CARTESIAN_POINT('Ctrl Pts',(-13.2302726269444,-4.98245867427902,
0.405600937068007));
#12835=CARTESIAN_POINT('Ctrl Pts',(-13.2505381529841,-4.98245867427902,
-0.68247630754827));
#12836=CARTESIAN_POINT('Origin',(-13.5749885148034,2.62967685638955,-4.46806532836687));
#12837=CARTESIAN_POINT('',(-16.497528189245,-2.87032314361045,-1.54552565392526));
#12838=CARTESIAN_POINT('',(-13.5749885148034,-2.87032314361045,-4.46806532836687));
#12839=CARTESIAN_POINT('',(-16.497528189245,2.62967685638955,-1.54552565392526));
#12840=CARTESIAN_POINT('Origin',(-21.3531631078554,-2.87032314361045,-12.2462399214189));
#12841=CARTESIAN_POINT('',(-14.9418932706346,-2.87032314361045,-1.54552565392526));
#12842=CARTESIAN_POINT('',(-19.6087980264659,-2.87032314361045,-6.21243040975647));
#12843=CARTESIAN_POINT('Origin',(-15.7197107299398,-2.87032314361045,-0.767708194620052));
#12844=CARTESIAN_POINT('Origin',(-21.3531631078554,2.62967685638955,-12.2462399214189));
#12845=CARTESIAN_POINT('',(-16.497528189245,2.62967685638955,-1.54552565392526));
#12846=CARTESIAN_POINT('',(-13.5749885148034,2.62967685638955,-4.46806532836687));
#12847=CARTESIAN_POINT('',(-14.9418932706346,2.62967685638955,-1.54552565392526));
#12848=CARTESIAN_POINT('',(-19.6087980264659,2.62967685638955,-6.21243040975647));
#12849=CARTESIAN_POINT('Origin',(-15.7197107299398,2.62967685638955,-0.767708194620052));
#12850=CARTESIAN_POINT('Origin',(-12.0361190763098,0.000349899298694283,
-13.7851093599125));
#12851=CARTESIAN_POINT('',(-20.3866154857711,-4.98245867427902,-5.43461295045127));
#12852=CARTESIAN_POINT('',(-22.1309805671606,-4.98245867427902,-3.69024786906167));
#12853=CARTESIAN_POINT('',(-19.6087980264659,-4.98245867427902,-6.21243040975647));
#12854=CARTESIAN_POINT('',(-22.1309805671606,-2.87032314361045,-3.69024786906167));
#12855=CARTESIAN_POINT('',(-22.1309805671606,-2.87032314361045,-3.69024786906167));
#12856=CARTESIAN_POINT('',(-20.3866154857711,-2.87032314361045,-5.43461295045127));
#12857=CARTESIAN_POINT('',(-12.0361190763098,-2.87032314361045,-13.7851093599125));
#12858=CARTESIAN_POINT('',(-20.3866154857711,-4.98245867427902,-5.43461295045127));
#12859=CARTESIAN_POINT('Origin',(0.135922068665986,0.000349899298694283,
-1.61306821493671));
#12860=CARTESIAN_POINT('',(-13.3395039193314,-4.74107350453719,-0.767708194620046));
#12861=CARTESIAN_POINT('Origin',(0.135922068665986,0.000349899298694283,
-0.767708194620051));
#12862=CARTESIAN_POINT('Ctrl Pts',(-13.3395039193314,-4.74107350453718,
-0.767708194620051));
#12863=CARTESIAN_POINT('Ctrl Pts',(-13.5595899825791,-4.12673469180454,
-0.979912166561785));
#12864=CARTESIAN_POINT('Ctrl Pts',(-13.7382816024804,-3.49326423992937,
-1.16221207358175));
#12865=CARTESIAN_POINT('Ctrl Pts',(-14.0655382696254,-1.91389512029188,
-1.50346894589392));
#12866=CARTESIAN_POINT('Ctrl Pts',(-14.164077931334,-0.954643474757865,
-1.61306821493671));
#12867=CARTESIAN_POINT('Ctrl Pts',(-14.164077931334,0.955343273355252,-1.61306821493671));
#12868=CARTESIAN_POINT('Ctrl Pts',(-14.0655382696254,1.91459491888927,-1.50346894589392));
#12869=CARTESIAN_POINT('Ctrl Pts',(-13.7382816024804,3.49396403852676,-1.16221207358175));
#12870=CARTESIAN_POINT('Ctrl Pts',(-13.5595899825791,4.12743449040194,-0.979912166561781));
#12871=CARTESIAN_POINT('Ctrl Pts',(-13.3395039193314,4.74177330313459,-0.767708194620044));
#12872=CARTESIAN_POINT('Origin',(0.0218920916114575,39.6003498992987,-14.6253990787018));
#12873=CARTESIAN_POINT('',(-8.66407793133402,-8.24965010070131,2.55355388009327));
#12874=CARTESIAN_POINT('',(-5.0804571785076,-8.24965010070131,3.93608070944324));
#12875=CARTESIAN_POINT('Origin',(0.0218920916114575,-8.24965010070131,-14.6253990787018));
#12876=CARTESIAN_POINT('',(-5.0804571785076,39.6003498992987,3.93608070944324));
#12877=CARTESIAN_POINT('Origin',(-3.56182917946212,1.09754136743265,5.99267018676129));
#12878=CARTESIAN_POINT('',(-5.0804571785076,8.25034989929869,3.93608070944324));
#12879=CARTESIAN_POINT('',(-5.0804571785076,39.6003498992987,3.93608070944324));
#12880=CARTESIAN_POINT('',(-8.66407793133402,8.25034989929869,2.55355388009326));
#12881=CARTESIAN_POINT('Origin',(0.0218920916114575,8.2503498992987,-14.6253990787018));
#12882=CARTESIAN_POINT('',(-8.66407793133402,39.6003498992987,2.55355388009327));
#12883=CARTESIAN_POINT('Origin',(14.2061209221522,39.6003498992987,-1.45654689569859));
#12884=CARTESIAN_POINT('',(13.9997902889911,-17.,17.0911694938297));
#12885=CARTESIAN_POINT('',(13.9019434616744,0.000349899298694283,25.8869317850633));
#12886=CARTESIAN_POINT('Origin',(0.135922068665986,0.000349899298694283,
25.8869317850633));
#12887=CARTESIAN_POINT('Origin',(17.735922068666,-8.24965010070131,-16.9581329720854));
#12888=CARTESIAN_POINT('',(-0.11761019287632,-8.24965010070131,7.09490065582709));
#12889=CARTESIAN_POINT('',(7.42524145690086,-8.24965010070131,13.731996542212));
#12890=CARTESIAN_POINT('Origin',(26.5767111010661,-8.24965010070131,-15.6377043248233));
#12891=CARTESIAN_POINT('Origin',(-7.7310282279201,-8.24965010070131,13.578407872116));
#12892=CARTESIAN_POINT('',(-8.66407793133402,-8.24965010070131,21.731996542212));
#12893=CARTESIAN_POINT('',(-8.66407793133402,-8.24965010070131,-16.9581329720854));
#12894=CARTESIAN_POINT('',(7.42524145690086,-8.24965010070131,21.731996542212));
#12895=CARTESIAN_POINT('',(7.42524145690086,-8.24965010070131,21.731996542212));
#12896=CARTESIAN_POINT('',(7.42524145690086,-8.24965010070131,21.731996542212));
#12897=CARTESIAN_POINT('Origin',(17.735922068666,8.2503498992987,-16.9581329720854));
#12898=CARTESIAN_POINT('',(-0.11761019287632,8.25034989929869,7.09490065582709));
#12899=CARTESIAN_POINT('Origin',(-7.7310282279201,8.25034989929869,13.578407872116));
#12900=CARTESIAN_POINT('',(7.42524145690086,8.25034989929869,13.731996542212));
#12901=CARTESIAN_POINT('Origin',(26.5767111010661,8.2503498992987,-15.6377043248233));
#12902=CARTESIAN_POINT('',(7.42524145690086,8.25034989929869,21.731996542212));
#12903=CARTESIAN_POINT('',(7.42524145690086,8.25034989929869,21.731996542212));
#12904=CARTESIAN_POINT('',(-8.66407793133402,8.25034989929869,21.731996542212));
#12905=CARTESIAN_POINT('',(-8.66407793133402,8.25034989929869,21.731996542212));
#12906=CARTESIAN_POINT('',(-8.66407793133402,8.2503498992987,-16.9581329720854));
#12907=CARTESIAN_POINT('Origin',(-8.66407793133402,0.000349899298694283,
-1.61306821493671));
#12908=CARTESIAN_POINT('',(-8.66407793133402,-8.24965010070131,21.731996542212));
#12909=CARTESIAN_POINT('Origin',(14.2231693005462,-4.98245867427902,-0.767708194620051));
#12910=CARTESIAN_POINT('',(-13.2521255922709,-4.98245867427902,-0.767708194620051));
#12911=CARTESIAN_POINT('Origin',(0.135922068665986,0.000349899298694283,
-0.767708194620051));
#12912=CARTESIAN_POINT('',(-14.1640758113294,-4.98245867427902,-0.76770819462005));
#12913=CARTESIAN_POINT('',(14.2231693005462,-4.98245867427902,-0.767708194620051));
#12914=CARTESIAN_POINT('',(-14.1640758113294,4.74181238705812,-0.767708194620056));
#12915=CARTESIAN_POINT('',(-14.1640758113294,-4.98245867427902,-0.767708194620051));
#12916=CARTESIAN_POINT('',(14.2231693005462,4.74181238705812,-0.767708194620051));
#12917=CARTESIAN_POINT('Origin',(14.2231693005462,4.74181238705812,5.83229180537995));
#12918=CARTESIAN_POINT('',(-22.1309805671606,4.74181238705812,-3.69024786906167));
#12919=CARTESIAN_POINT('',(-20.386615485771,4.74181238705812,-5.43461295045127));
#12920=CARTESIAN_POINT('',(-22.9087980264659,4.74181238705812,-2.91243040975647));
#12921=CARTESIAN_POINT('',(-22.1309805671606,4.74181238705812,-2.13461295045127));
#12922=CARTESIAN_POINT('Origin',(-21.3531631078554,4.74181238705812,-2.91243040975647));
#12923=CARTESIAN_POINT('',(-14.1640758113294,4.74181238705812,5.83229180537995));
#12924=CARTESIAN_POINT('',(-22.9087980264659,4.74181238705812,-2.91243040975647));
#12925=CARTESIAN_POINT('',(14.2231693005462,4.74181238705812,5.83229180537995));
#12926=CARTESIAN_POINT('',(-18.8309805671606,4.74181238705812,-5.43461295045127));
#12927=CARTESIAN_POINT('',(-19.6087980264659,4.74181238705812,-6.21243040975647));
#12928=CARTESIAN_POINT('Origin',(-19.6087980264659,4.74181238705812,-4.65679549114606));
#12929=CARTESIAN_POINT('Origin',(14.2231693005462,-4.98245867427902,5.83229180537995));
#12930=CARTESIAN_POINT('',(-14.1640758113294,-4.98245867427902,5.83229180537995));
#12931=CARTESIAN_POINT('',(-14.1640758113294,-4.98245867427902,5.83229180537995));
#12932=CARTESIAN_POINT('',(14.2231693005462,-4.98245867427902,5.83229180537995));
#12933=CARTESIAN_POINT('Origin',(14.2231693005462,-4.98245867427902,5.83229180537995));
#12934=CARTESIAN_POINT('',(-22.1309805671606,-4.98245867427902,-2.13461295045127));
#12935=CARTESIAN_POINT('',(-22.9087980264659,-4.98245867427902,-2.91243040975647));
#12936=CARTESIAN_POINT('Origin',(-21.3531631078554,-4.98245867427902,-2.91243040975647));
#12937=CARTESIAN_POINT('',(-18.8309805671606,-4.98245867427902,-5.43461295045127));
#12938=CARTESIAN_POINT('Origin',(-19.6087980264659,-4.98245867427902,-4.65679549114606));
#12939=CARTESIAN_POINT('',(-19.6087980264659,-4.98245867427902,-6.21243040975647));
#12940=CARTESIAN_POINT('',(-13.2505381529841,-4.98245867427902,-0.68247630754827));
#12941=CARTESIAN_POINT('Origin',(0.135922068665986,0.000349899298694283,
-1.61306821493671));
#12942=CARTESIAN_POINT('Origin',(-19.6087980264659,4.74181238705812,-6.21243040975647));
#12943=CARTESIAN_POINT('',(-18.8309805671606,2.62967685638955,-5.43461295045127));
#12944=CARTESIAN_POINT('',(-19.6087980264659,2.62967685638955,-6.21243040975647));
#12945=CARTESIAN_POINT('',(-18.8309805671606,4.74181238705812,-5.43461295045127));
#12946=CARTESIAN_POINT('',(-18.8309805671606,-2.87032314361045,-5.43461295045127));
#12947=CARTESIAN_POINT('',(-18.8309805671606,-2.87032314361045,-5.43461295045127));
#12948=CARTESIAN_POINT('',(-19.6087980264659,-2.87032314361045,-6.21243040975647));
#12949=CARTESIAN_POINT('',(-14.9418932706346,4.74181238705812,-1.54552565392526));
#12950=CARTESIAN_POINT('Origin',(-22.9087980264659,-4.98245867427902,-2.91243040975647));
#12951=CARTESIAN_POINT('',(-22.1309805671606,2.62967685638955,-2.13461295045127));
#12952=CARTESIAN_POINT('',(-26.7978853229919,2.62967685638955,-6.80151770628248));
#12953=CARTESIAN_POINT('',(-22.1309805671606,-2.87032314361045,-2.13461295045127));
#12954=CARTESIAN_POINT('',(-26.7978853229919,-2.87032314361045,-6.80151770628248));
#12955=CARTESIAN_POINT('',(-22.1309805671606,-4.98245867427902,-2.13461295045127));
#12956=CARTESIAN_POINT('',(-22.1309805671606,2.62967685638955,-2.13461295045127));
#12957=CARTESIAN_POINT('Origin',(-12.0361190763098,0.000349899298694283,
-13.7851093599125));
#12958=CARTESIAN_POINT('',(-22.1309805671606,2.62967685638955,-3.69024786906167));
#12959=CARTESIAN_POINT('',(-20.3866154857711,2.62967685638955,-5.43461295045127));
#12960=CARTESIAN_POINT('',(-12.0361190763098,2.62967685638955,-13.7851093599125));
#12961=CARTESIAN_POINT('',(-22.1309805671606,4.74181238705812,-3.69024786906167));
#12962=CARTESIAN_POINT('',(-20.3866154857711,2.62967685638955,-5.43461295045127));
#12963=CARTESIAN_POINT('Origin',(-13.5749885148034,2.62967685638955,-4.46806532836687));
#12964=CARTESIAN_POINT('',(-16.497528189245,2.62967685638955,-1.54552565392526));
#12965=CARTESIAN_POINT('Origin',(-21.3531631078554,-2.87032314361045,-12.2462399214189));
#12966=CARTESIAN_POINT('Origin',(-19.6087980264659,-2.87032314361045,-4.65679549114606));
#12967=CARTESIAN_POINT('Origin',(-21.3531631078554,-2.87032314361045,-2.91243040975647));
#12968=CARTESIAN_POINT('Origin',(-21.3531631078554,2.62967685638955,-12.2462399214189));
#12969=CARTESIAN_POINT('Origin',(-21.3531631078554,2.62967685638955,-2.91243040975647));
#12970=CARTESIAN_POINT('Origin',(-19.6087980264659,2.62967685638955,-4.65679549114606));
#12971=CARTESIAN_POINT('Origin',(-19.7031631078554,-6.08245867427902,-3.00679549114607));
#12972=CARTESIAN_POINT('Origin',(-19.7031631078554,5.84154132572098,-3.00679549114607));
#12973=CARTESIAN_POINT('Origin',(-21.3531631078554,0.000349899298694283,
-2.91243040975647));
#12974=CARTESIAN_POINT('Origin',(-21.3531631078554,0.000349899298694283,
-2.91243040975647));
#12975=CARTESIAN_POINT('Origin',(-19.6087980264659,0.000349899298694283,
-4.65679549114606));
#12976=CARTESIAN_POINT('Origin',(-19.6087980264659,0.000349899298694283,
-4.65679549114606));
#12977=CARTESIAN_POINT('Origin',(-15.7197107299398,4.74181238705812,-0.767708194620052));
#12978=CARTESIAN_POINT('Origin',(26.5767111010661,-17.,-15.6377043248233));
#12979=CARTESIAN_POINT('',(-0.11761019287632,-17.,7.09490065582709));
#12980=CARTESIAN_POINT('',(7.42524145690086,-17.,13.731996542212));
#12981=CARTESIAN_POINT('',(-0.11761019287632,-17.,7.09490065582709));
#12982=CARTESIAN_POINT('Origin',(7.42524145690086,8.25034989929869,21.731996542212));
#12983=CARTESIAN_POINT('',(7.42524145690086,8.25034989929869,21.731996542212));
#12984=CARTESIAN_POINT('Origin',(-6.22633625589568E-31,-3.81260606886127E-15,
21.731996542212));
#12985=CARTESIAN_POINT('Origin',(-7.7310282279201,39.6003498992987,13.578407872116));
#12986=CARTESIAN_POINT('Origin',(-7.7310282279201,39.6003498992987,13.578407872116));
#13168=UNCERTAINTY_MEASURE_WITH_UNIT(LENGTH_MEASURE(0.01),#13200,
'DISTANCE_ACCURACY_VALUE',
'Maximum model space distance between geometric entities at asserted c
onnectivities');
#13173=UNCERTAINTY_MEASURE_WITH_UNIT(LENGTH_MEASURE(0.01),#13200,
'DISTANCE_ACCURACY_VALUE',
'Maximum model space distance between geometric entities at asserted c
onnectivities');
#13194=(
GEOMETRIC_REPRESENTATION_CONTEXT(3)
GLOBAL_UNCERTAINTY_ASSIGNED_CONTEXT((#13168))
GLOBAL_UNIT_ASSIGNED_CONTEXT((#13200,#13202,#13203))
REPRESENTATION_CONTEXT('','3D')
);
#13199=(
GEOMETRIC_REPRESENTATION_CONTEXT(3)
GLOBAL_UNCERTAINTY_ASSIGNED_CONTEXT((#13173))
GLOBAL_UNIT_ASSIGNED_CONTEXT((#13200,#13202,#13203))
REPRESENTATION_CONTEXT('','3D')
);
#13200=(
LENGTH_UNIT()
NAMED_UNIT(*)
SI_UNIT(.MILLI.,.METRE.)
);
#13202=(
NAMED_UNIT(*)
PLANE_ANGLE_UNIT()
SI_UNIT($,.RADIAN.)
);
#13203=(
NAMED_UNIT(*)
SI_UNIT($,.STERADIAN.)
SOLID_ANGLE_UNIT()
);
#13224=SHAPE_DEFINITION_REPRESENTATION(#13263,#13298);
#13263=PRODUCT_DEFINITION_SHAPE('',$,#13324);
#13298=SHAPE_REPRESENTATION('',(#7700),#13194);
#13303=PRODUCT_DEFINITION_CONTEXT('part definition',#13380,'design');
#13324=PRODUCT_DEFINITION('Thumb Link 2','Thumb Link 2',#13349,#13303);
#13349=PRODUCT_DEFINITION_FORMATION('',$,#13402);
#13380=APPLICATION_CONTEXT(
'Core Data for Automotive Mechanical Design Process');
#13381=PRODUCT_CONTEXT('part definition',#13380,'mechanical');
#13402=PRODUCT('Thumb Link 2','Thumb Link 2',$,(#13381));
#13409=PRESENTATION_STYLE_ASSIGNMENT((#13414));
#13414=SURFACE_STYLE_USAGE(.BOTH.,#13419);
#13419=SURFACE_SIDE_STYLE('',(#13424));
#13424=SURFACE_STYLE_FILL_AREA(#13429);
#13429=FILL_AREA_STYLE('Opaque(61,176,222)',(#13434));
#13434=FILL_AREA_STYLE_COLOUR('Opaque(61,176,222)',#13439);
#13439=COLOUR_RGB('Opaque(61,176,222)',0.23921568627451,0.690196078431373,
0.870588235294118);
ENDSEC;
END-ISO-10303-21;
